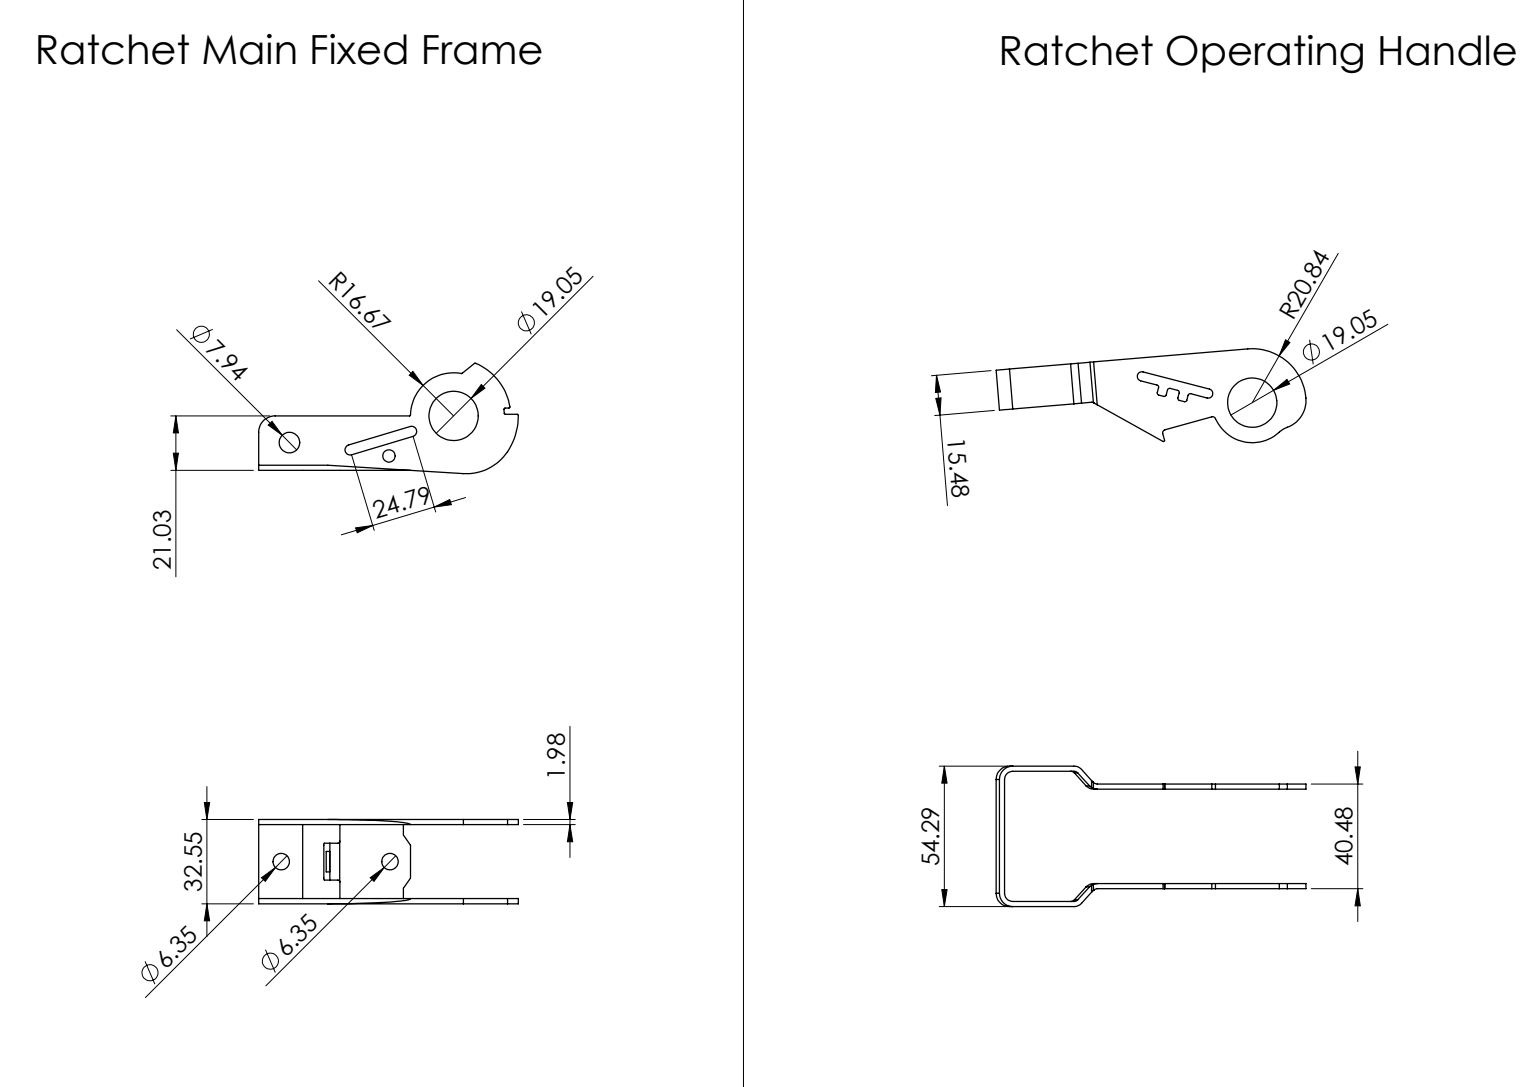
ISO-10303-21;
HEADER;
FILE_DESCRIPTION (('STEP AP214'),
    '1' );
FILE_NAME ('Ratchet Operating Handle.step',
    '2026-10-09T14:10:49',
    ( '' ),
    ( '' ),
    'SwSTEP 2.0',
    'SolidWorks 2026',
    '' );
FILE_SCHEMA (( 'AUTOMOTIVE_DESIGN' ));
ENDSEC;

DATA;
#1=VERTEX_POINT ( 'NONE', #18707 ) ;
#21=PLANE ( 'NONE',  #4977 ) ;
#37=EDGE_CURVE ( 'NONE', #10557, #1153, #11768, .T. ) ;
#54=VECTOR ( 'NONE', #11480, 1000.000000000000000 ) ;
#57=VECTOR ( 'NONE', #329, 1000.000000000000114 ) ;
#69=DIRECTION ( 'NONE',  ( -0.000000000000000000, -1.000000000000000000, 0.000000000000000000 ) ) ;
#81=LINE ( 'NONE', #19981, #4674 ) ;
#82=CARTESIAN_POINT ( 'NONE',  ( 29.01020070778135818, -3.968114999999999615, -13.85841188422236492 ) ) ;
#84=DIRECTION ( 'NONE',  ( 0.000000000000000000, 1.000000000000000000, 0.000000000000000000 ) ) ;
#85=CARTESIAN_POINT ( 'NONE',  ( -47.86112874365709047, 43.41875999999999891, -23.29368419115692035 ) ) ;
#88=ADVANCED_FACE ( 'NONE', ( #14317 ), #12096, .F. ) ;
#113=EDGE_LOOP ( 'NONE', ( #12441, #427, #14936, #388, #14608 ) ) ;
#128=VECTOR ( 'NONE', #842, 1000.000000000000000 ) ;
#135=VECTOR ( 'NONE', #21119, 1000.000000000000000 ) ;
#136=CARTESIAN_POINT ( 'NONE',  ( 20.56513292926062775, -14.84248999999999974, -10.49765270116350280 ) ) ;
#144=LINE ( 'NONE', #10317, #14114 ) ;
#149=EDGE_CURVE ( 'NONE', #1153, #19768, #10533, .T. ) ;
#153=VECTOR ( 'NONE', #12221, 1000.000000000000114 ) ;
#171=VERTEX_POINT ( 'NONE', #19036 ) ;
#172=DIRECTION ( 'NONE',  ( 0.000000000000000000, 1.000000000000000000, 0.000000000000000000 ) ) ;
#178=ORIENTED_EDGE ( 'NONE', *, *, #11385, .F. ) ;
#179=DIRECTION ( 'NONE',  ( -0.2490110332224836354, 0.000000000000000000, 0.9685006480810794960 ) ) ;
#193=( NAMED_UNIT ( * ) PLANE_ANGLE_UNIT ( ) SI_UNIT ( $, .RADIAN. ) );
#201=LINE ( 'NONE', #6943, #11370 ) ;
#211=ADVANCED_FACE ( 'NONE', ( #17509 ), #9084, .T. ) ;
#212=EDGE_CURVE ( 'NONE', #18633, #13378, #14563, .T. ) ;
#216=CARTESIAN_POINT ( 'NONE',  ( 19.79515554403045741, -1.983739999999999393, -10.69562145279641996 ) ) ;
#227=VERTEX_POINT ( 'NONE', #17942 ) ;
#236=CARTESIAN_POINT ( 'NONE',  ( -24.21104940531825633, 39.44874000000000080, -25.29232732678598339 ) ) ;
#246=CYLINDRICAL_SURFACE ( 'NONE', #5483, 3.970019999999997662 ) ;
#254=DIRECTION ( 'NONE',  ( -0.000000000000000000, -1.000000000000000000, 0.000000000000000000 ) ) ;
#255=PLANE ( 'NONE',  #7057 ) ;
#256=ORIENTED_EDGE ( 'NONE', *, *, #13831, .T. ) ;
#258=CARTESIAN_POINT ( 'NONE',  ( -13.87747867115857936, -3.968114999999999615, -9.458632424640695646 ) ) ;
#269=DIRECTION ( 'NONE',  ( -0.9685006480810792739, 0.000000000000000000, -0.2490110332224846346 ) ) ;
#276=EDGE_LOOP ( 'NONE', ( #21374, #11121, #4887, #17818 ) ) ;
#277=DIRECTION ( 'NONE',  ( 0.9964481331860212121, 0.000000000000000000, -0.08420877549337300871 ) ) ;
#283=DIRECTION ( 'NONE',  ( 0.7334850928793773539, -0.6768732144311023768, -0.06198604769976986950 ) ) ;
#287=CARTESIAN_POINT ( 'NONE',  ( 18.07371581377308800, 36.51313500000000545, -11.95909761906105473 ) ) ;
#296=CIRCLE ( 'NONE', #18309, 1.983739999999999393 ) ;
#298=DIRECTION ( 'NONE',  ( -0.4857267349359786768, 0.000000000000000000, 0.8741107132214052111 ) ) ;
#317=AXIS2_PLACEMENT_3D ( 'NONE', #448, #20660, #3437 ) ;
#329=DIRECTION ( 'NONE',  ( -0.9685006480810792739, 0.000000000000000000, -0.2490110332224846346 ) ) ;
#336=EDGE_CURVE ( 'NONE', #2732, #10479, #8823, .T. ) ;
#337=VERTEX_POINT ( 'NONE', #7187 ) ;
#338=CARTESIAN_POINT ( 'NONE',  ( -15.39353573898878658, -2.254660308866960339, -10.30107656633069979 ) ) ;
#339=EDGE_CURVE ( 'NONE', #11891, #20381, #4666, .T. ) ;
#345=DIRECTION ( 'NONE',  ( 0.000000000000000000, 1.000000000000000000, 0.000000000000000000 ) ) ;
#352=AXIS2_PLACEMENT_3D ( 'NONE', #14843, #6560, #1786 ) ;
#355=DIRECTION ( 'NONE',  ( 0.2490110332224846623, 0.000000000000000000, -0.9685006480810793850 ) ) ;
#358=CARTESIAN_POINT ( 'NONE',  ( 12.25799425556778388, 34.52875999999999834, 0.2069032437451798767 ) ) ;
#362=EDGE_CURVE ( 'NONE', #10171, #5161, #12705, .T. ) ;
#366=CARTESIAN_POINT ( 'NONE',  ( -53.00154558624916490, -5.714999999999999858, -22.85927301266823264 ) ) ;
#369=DIRECTION ( 'NONE',  ( -0.9964481331860212121, 0.000000000000000000, 0.08420877549337300871 ) ) ;
#374=VERTEX_POINT ( 'NONE', #3870 ) ;
#382=VECTOR ( 'NONE', #11141, 1000.000000000000000 ) ;
#383=CARTESIAN_POINT ( 'NONE',  ( 17.10576967688479399, -14.84248999999999974, -11.38708898545455561 ) ) ;
#385=ORIENTED_EDGE ( 'NONE', *, *, #5454, .T. ) ;
#388=ORIENTED_EDGE ( 'NONE', *, *, #17748, .F. ) ;
#397=AXIS2_PLACEMENT_3D ( 'NONE', #13888, #8758, #15657 ) ;
#398=DIRECTION ( 'NONE',  ( 0.4857267349359797870, 0.000000000000000000, -0.8741107132214044340 ) ) ;
#403=CARTESIAN_POINT ( 'NONE',  ( 29.45491884992628329, 34.52875999999999834, -15.58809351040512325 ) ) ;
#407=VECTOR ( 'NONE', #5440, 1000.000000000000000 ) ;
#414=CARTESIAN_POINT ( 'NONE',  ( 17.22522857595987844, 34.52875999999999834, -15.04442098945225403 ) ) ;
#422=AXIS2_PLACEMENT_3D ( 'NONE', #16207, #16521, #8217 ) ;
#427=ORIENTED_EDGE ( 'NONE', *, *, #17403, .F. ) ;
#428=ORIENTED_EDGE ( 'NONE', *, *, #17879, .F. ) ;
#437=EDGE_CURVE ( 'NONE', #16850, #6939, #17013, .T. ) ;
#438=CARTESIAN_POINT ( 'NONE',  ( 31.83819605565793509, 34.52875999999999834, -4.158220719828246814 ) ) ;
#443=ORIENTED_EDGE ( 'NONE', *, *, #13997, .T. ) ;
#445=CARTESIAN_POINT ( 'NONE',  ( 17.87574706213523612, -3.968114999999999615, -11.18912023382283571 ) ) ;
#446=DIRECTION ( 'NONE',  ( -0.2490110332224846346, 0.000000000000000000, 0.9685006480810792739 ) ) ;
#448=CARTESIAN_POINT ( 'NONE',  ( 55.81697695389291169, -14.84248999999999974, -11.14520323105768362 ) ) ;
#451=ADVANCED_FACE ( 'NONE', ( #15819 ), #9149, .F. ) ;
#458=ORIENTED_EDGE ( 'NONE', *, *, #17617, .T. ) ;
#460=CARTESIAN_POINT ( 'NONE',  ( -15.84035234298960049, -2.442431200715369677, -10.46642885967791692 ) ) ;
#464=CARTESIAN_POINT ( 'NONE',  ( 11.56192577415882816, -1.983739999999999393, 4.677561850332325299 ) ) ;
#466=DIRECTION ( 'NONE',  ( -0.4857267349359799535, 0.000000000000000000, 0.8741107132214044340 ) ) ;
#471=PRODUCT_DEFINITION ( 'UNKNOWN', '', #9128, #21835 ) ;
#487=DIRECTION ( 'NONE',  ( -0.2490110332224846346, 0.000000000000000000, 0.9685006480810792739 ) ) ;
#488=AXIS2_PLACEMENT_3D ( 'NONE', #287, #69, #10464 ) ;
#489=DIRECTION ( 'NONE',  ( -0.9685006480810794960, 0.000000000000000000, -0.2490110332224836354 ) ) ;
#496=EDGE_CURVE ( 'NONE', #17843, #3371, #1299, .T. ) ;
#519=ADVANCED_FACE ( 'NONE', ( #14481 ), #16142, .F. ) ;
#520=CARTESIAN_POINT ( 'NONE',  ( 46.03750000000000142, -14.84248999999999974, -10.31874999999999964 ) ) ;
#534=DIRECTION ( 'NONE',  ( 0.7334850928793772429, -0.6768732144311024879, -0.06198604769977036216 ) ) ;
#545=CARTESIAN_POINT ( 'NONE',  ( 46.03750000000000142, -3.968114999999999615, -10.31874999999999964 ) ) ;
#549=ORIENTED_EDGE ( 'NONE', *, *, #989, .F. ) ;
#552=LINE ( 'NONE', #7622, #13154 ) ;
#555=DIRECTION ( 'NONE',  ( 0.000000000000000000, 1.000000000000000000, 0.000000000000000000 ) ) ;
#556=ADVANCED_FACE ( 'NONE', ( #9374 ), #2746, .T. ) ;
#558=ORIENTED_EDGE ( 'NONE', *, *, #17949, .F. ) ;
#561=CARTESIAN_POINT ( 'NONE',  ( 22.02657784715807665, 128.5105379999999968, -12.98906981665815330 ) ) ;
#579=DIRECTION ( 'NONE',  ( -0.9964481331860213231, 0.000000000000000000, 0.08420877549337293932 ) ) ;
#586=ORIENTED_EDGE ( 'NONE', *, *, #10826, .T. ) ;
#590=ORIENTED_EDGE ( 'NONE', *, *, #21010, .F. ) ;
#595=ORIENTED_EDGE ( 'NONE', *, *, #11225, .F. ) ;
#601=FACE_OUTER_BOUND ( 'NONE', #956, .T. ) ;
#605=ORIENTED_EDGE ( 'NONE', *, *, #6499, .F. ) ;
#608=DIRECTION ( 'NONE',  ( 0.08420877549337300871, 0.000000000000000000, 0.9964481331860212121 ) ) ;
#612=CARTESIAN_POINT ( 'NONE',  ( 3.805353748838121053, -1.983739999999999393, -22.18284873352824960 ) ) ;
#615=ORIENTED_EDGE ( 'NONE', *, *, #14572, .T. ) ;
#618=ADVANCED_FACE ( 'NONE', ( #9701 ), #12829, .F. ) ;
#626=CARTESIAN_POINT ( 'NONE',  ( 17.99520596118501814, -14.84248999999999974, -14.84645223781840073 ) ) ;
#627=FACE_OUTER_BOUND ( 'NONE', #9472, .T. ) ;
#639=EDGE_CURVE ( 'NONE', #5833, #5959, #21527, .T. ) ;
#649=CARTESIAN_POINT ( 'NONE',  ( 11.42842559562532578, -3.968114999999999615, 1.673196738795719174 ) ) ;
#657=ORIENTED_EDGE ( 'NONE', *, *, #6799, .T. ) ;
#660=DIRECTION ( 'NONE',  ( 0.2490110332224846346, 0.000000000000000000, -0.9685006480810792739 ) ) ;
#666=LINE ( 'NONE', #20779, #7420 ) ;
#674=EDGE_CURVE ( 'NONE', #1, #6701, #6424, .T. ) ;
#680=AXIS2_PLACEMENT_3D ( 'NONE', #2628, #20743, #5925 ) ;
#686=FACE_OUTER_BOUND ( 'NONE', #17221, .T. ) ;
#694=CARTESIAN_POINT ( 'NONE',  ( -16.14706788831979978, 36.51313500000000545, -25.97380585690919830 ) ) ;
#698=CARTESIAN_POINT ( 'NONE',  ( 28.56548256563643662, -14.84248999999999974, -12.12873025803960658 ) ) ;
#701=AXIS2_PLACEMENT_3D ( 'NONE', #14633, #10960, #2564 ) ;
#714=ORIENTED_EDGE ( 'NONE', *, *, #19357, .F. ) ;
#722=LINE ( 'NONE', #20832, #16647 ) ;
#725=CYLINDRICAL_SURFACE ( 'NONE', #8862, 20.83593749999999289 ) ;
#728=DIRECTION ( 'NONE',  ( 0.000000000000000000, 1.000000000000000000, 0.000000000000000000 ) ) ;
#737=CARTESIAN_POINT ( 'NONE',  ( -46.55773479047372376, 43.41875999999999891, -7.870535429687039120 ) ) ;
#740=ORIENTED_EDGE ( 'NONE', *, *, #20509, .F. ) ;
#742=VECTOR ( 'NONE', #16555, 1000.000000000000114 ) ;
#755=AXIS2_PLACEMENT_3D ( 'NONE', #8975, #21028, #5874 ) ;
#759=CYLINDRICAL_SURFACE ( 'NONE', #18143, 3.970019999999997662 ) ;
#779=ORIENTED_EDGE ( 'NONE', *, *, #14955, .F. ) ;
#785=CARTESIAN_POINT ( 'NONE',  ( 12.13621795668766445, 36.51313500000000545, 4.225309685850866082 ) ) ;
#800=PLANE ( 'NONE',  #15930 ) ;
#801=FACE_OUTER_BOUND ( 'NONE', #18130, .T. ) ;
#823=ADVANCED_FACE ( 'NONE', ( #18322 ), #1521, .F. ) ;
#828=ORIENTED_EDGE ( 'NONE', *, *, #12493, .F. ) ;
#842=DIRECTION ( 'NONE',  ( 0.000000000000000000, 1.000000000000000000, 0.000000000000000000 ) ) ;
#846=ORIENTED_EDGE ( 'NONE', *, *, #8565, .F. ) ;
#848=CARTESIAN_POINT ( 'NONE',  ( -15.27935546639805331, -3.968114999999999615, -26.04713531390440906 ) ) ;
#853=CARTESIAN_POINT ( 'NONE',  ( 21.25660046192028929, -3.968114999999999615, -13.18703856829094079 ) ) ;
#870=ORIENTED_EDGE ( 'NONE', *, *, #639, .T. ) ;
#882=EDGE_CURVE ( 'NONE', #20855, #10784, #15692, .T. ) ;
#889=ORIENTED_EDGE ( 'NONE', *, *, #967, .T. ) ;
#898=ADVANCED_FACE ( 'NONE', ( #17208 ), #2170, .T. ) ;
#899=ADVANCED_FACE ( 'NONE', ( #19304 ), #7270, .T. ) ;
#902=CARTESIAN_POINT ( 'NONE',  ( 62.90077106633562209, -1.983739999999999393, 8.141649473166729933 ) ) ;
#919=ORIENTED_EDGE ( 'NONE', *, *, #7931, .T. ) ;
#920=CARTESIAN_POINT ( 'NONE',  ( 12.57635667311951622, -95.96551800000000298, 1.354834321244424267 ) ) ;
#932=DIRECTION ( 'NONE',  ( 0.9964481331860212121, 0.000000000000000000, -0.08420877549337300871 ) ) ;
#945=ORIENTED_EDGE ( 'NONE', *, *, #5714, .F. ) ;
#950=VECTOR ( 'NONE', #4203, 1000.000000000000000 ) ;
#951=DIRECTION ( 'NONE',  ( 0.08420877549337300871, 0.000000000000000000, 0.9964481331860212121 ) ) ;
#952=ORIENTED_EDGE ( 'NONE', *, *, #8551, .F. ) ;
#956=EDGE_LOOP ( 'NONE', ( #8354, #9146, #16354, #4398, #16333 ) ) ;
#957=ORIENTED_EDGE ( 'NONE', *, *, #13068, .F. ) ;
#967=EDGE_CURVE ( 'NONE', #10206, #3833, #5592, .T. ) ;
#969=DIRECTION ( 'NONE',  ( 0.2490110332224846623, 0.000000000000000000, -0.9685006480810793850 ) ) ;
#972=DIRECTION ( 'NONE',  ( 0.08420877549337300871, 0.000000000000000000, 0.9964481331860212121 ) ) ;
#987=ORIENTED_EDGE ( 'NONE', *, *, #21537, .F. ) ;
#988=CARTESIAN_POINT ( 'NONE',  ( 21.25660046192028929, 36.51313500000000545, -13.18703856829094079 ) ) ;
#989=EDGE_CURVE ( 'NONE', #17468, #15052, #4063, .T. ) ;
#997=LINE ( 'NONE', #1322, #15546 ) ;
#1029=AXIS2_PLACEMENT_3D ( 'NONE', #3066, #20273, #16870 ) ;
#1037=ORIENTED_EDGE ( 'NONE', *, *, #13043, .F. ) ;
#1054=VERTEX_POINT ( 'NONE', #6558 ) ;
#1064=CARTESIAN_POINT ( 'NONE',  ( 22.02657784715807665, 128.5105379999999968, -12.98906981665815330 ) ) ;
#1066=PLANE ( 'NONE',  #17926 ) ;
#1079=AXIS2_PLACEMENT_3D ( 'NONE', #9658, #1255, #20244 ) ;
#1080=DIRECTION ( 'NONE',  ( -0.7334850928793776870, -0.6768732144311018217, 0.06198604769977172219 ) ) ;
#1083=DIRECTION ( 'NONE',  ( 0.9964481331860213231, 0.000000000000000000, -0.08420877549337293932 ) ) ;
#1098=CARTESIAN_POINT ( 'NONE',  ( 13.28822531734660828, -3.968114999999999615, -15.23578611614444078 ) ) ;
#1102=CIRCLE ( 'NONE', #15593, 1.785937499999998179 ) ;
#1109=AXIS2_PLACEMENT_3D ( 'NONE', #9708, #17905, #16474 ) ;
#1122=ORIENTED_EDGE ( 'NONE', *, *, #16792, .F. ) ;
#1148=CARTESIAN_POINT ( 'NONE',  ( 56.47666780297049627, -3.968114999999999615, 1.109116340531466127 ) ) ;
#1153=VERTEX_POINT ( 'NONE', #3359 ) ;
#1155=DIRECTION ( 'NONE',  ( -0.9964481331860213231, 0.000000000000000000, 0.08420877549337311974 ) ) ;
#1178=VECTOR ( 'NONE', #4215, 1000.000000000000000 ) ;
#1189=CIRCLE ( 'NONE', #7538, 0.3962399999999998701 ) ;
#1203=DIRECTION ( 'NONE',  ( 0.2672484743474500268, 0.000000000000000000, 0.9636276526537417286 ) ) ;
#1205=CARTESIAN_POINT ( 'NONE',  ( 56.47666780297049627, -3.968114999999999615, 1.109116340531466127 ) ) ;
#1213=AXIS2_PLACEMENT_3D ( 'NONE', #19754, #4306, #16360 ) ;
#1230=LINE ( 'NONE', #7973, #13495 ) ;
#1238=VERTEX_POINT ( 'NONE', #1148 ) ;
#1246=CARTESIAN_POINT ( 'NONE',  ( 11.56192577415882816, 36.51313500000000545, 4.677561850332325299 ) ) ;
#1255=DIRECTION ( 'NONE',  ( 0.000000000000000000, -1.000000000000000000, 0.000000000000000000 ) ) ;
#1259=FACE_OUTER_BOUND ( 'NONE', #19368, .T. ) ;
#1270=ORIENTED_EDGE ( 'NONE', *, *, #10185, .T. ) ;
#1274=ORIENTED_EDGE ( 'NONE', *, *, #7778, .T. ) ;
#1297=CIRCLE ( 'NONE', #8709, 9.524999999999996803 ) ;
#1298=VERTEX_POINT ( 'NONE', #20448 ) ;
#1299=LINE ( 'NONE', #4515, #19490 ) ;
#1300=CARTESIAN_POINT ( 'NONE',  ( 3.360635606688116894, -14.84248999999999974, -20.45316710734507026 ) ) ;
#1309=CARTESIAN_POINT ( 'NONE',  ( 44.28293121686854761, -14.84248999999999974, -31.08068102505560759 ) ) ;
#1310=ORIENTED_EDGE ( 'NONE', *, *, #6278, .F. ) ;
#1314=VECTOR ( 'NONE', #9026, 1000.000000000000000 ) ;
#1318=EDGE_LOOP ( 'NONE', ( #8163, #16401, #5359, #8233 ) ) ;
#1322=CARTESIAN_POINT ( 'NONE',  ( 66.79943102505561114, 34.52875999999999834, -12.07331878313145168 ) ) ;
#1324=DIRECTION ( 'NONE',  ( -0.3447671952293630548, 0.000000000000000000, -0.9386882235831439658 ) ) ;
#1334=CARTESIAN_POINT ( 'NONE',  ( 11.82678039945931481, 34.52875999999999834, -12.74436900065013667 ) ) ;
#1339=ORIENTED_EDGE ( 'NONE', *, *, #14024, .F. ) ;
#1352=PLANE ( 'NONE',  #4444 ) ;
#1354=LINE ( 'NONE', #4474, #2136 ) ;
#1359=AXIS2_PLACEMENT_3D ( 'NONE', #18822, #254, #8753 ) ;
#1360=ORIENTED_EDGE ( 'NONE', *, *, #4217, .F. ) ;
#1367=ORIENTED_EDGE ( 'NONE', *, *, #16026, .F. ) ;
#1375=VERTEX_POINT ( 'NONE', #7425 ) ;
#1377=ADVANCED_FACE ( 'NONE', ( #19255 ), #5657, .F. ) ;
#1391=ORIENTED_EDGE ( 'NONE', *, *, #17921, .T. ) ;
#1392=CARTESIAN_POINT ( 'NONE',  ( 20.56513292926062775, -14.84248999999999974, -10.49765270116350280 ) ) ;
#1397=CIRCLE ( 'NONE', #21171, 0.7950200000000000600 ) ;
#1426=EDGE_LOOP ( 'NONE', ( #6037, #3965, #6020, #16638 ) ) ;
#1431=ADVANCED_FACE ( 'NONE', ( #7647 ), #14408, .T. ) ;
#1434=VECTOR ( 'NONE', #1830, 1000.000000000000114 ) ;
#1444=CARTESIAN_POINT ( 'NONE',  ( 12.13621795668766445, -3.968114999999999615, 4.225309685850866082 ) ) ;
#1447=CARTESIAN_POINT ( 'NONE',  ( -51.84716326864270286, -5.714364999999999029, -70.46824097531958842 ) ) ;
#1460=EDGE_CURVE ( 'NONE', #20489, #19935, #16020, .T. ) ;
#1468=DIRECTION ( 'NONE',  ( 0.2490110332224846623, 0.000000000000000000, -0.9685006480810793850 ) ) ;
#1478=DIRECTION ( 'NONE',  ( -0.9964481331860212121, 0.000000000000000000, 0.08420877549337300871 ) ) ;
#1490=ORIENTED_EDGE ( 'NONE', *, *, #10715, .F. ) ;
#1517=ADVANCED_FACE ( 'NONE', ( #19873 ), #19758, .T. ) ;
#1521=PLANE ( 'NONE',  #18095 ) ;
#1525=VERTEX_POINT ( 'NONE', #18125 ) ;
#1526=FACE_OUTER_BOUND ( 'NONE', #18731, .T. ) ;
#1530=VECTOR ( 'NONE', #12478, 1000.000000000000114 ) ;
#1532=ORIENTED_EDGE ( 'NONE', *, *, #17236, .T. ) ;
#1540=AXIS2_PLACEMENT_3D ( 'NONE', #3782, #466, #5769 ) ;
#1558=LINE ( 'NONE', #4877, #10288 ) ;
#1563=EDGE_CURVE ( 'NONE', #1054, #8841, #14380, .T. ) ;
#1564=EDGE_CURVE ( 'NONE', #21044, #4458, #13163, .T. ) ;
#1569=CARTESIAN_POINT ( 'NONE',  ( -15.39353573898878658, 34.79968030885680008, -10.30107656633069979 ) ) ;
#1570=AXIS2_PLACEMENT_3D ( 'NONE', #3806, #14001, #17411 ) ;
#1581=DIRECTION ( 'NONE',  ( -0.9685006480810793850, 0.000000000000000000, -0.2490110332224846623 ) ) ;
#1587=EDGE_CURVE ( 'NONE', #5833, #21613, #9486, .T. ) ;
#1622=VERTEX_POINT ( 'NONE', #21317 ) ;
#1624=DIRECTION ( 'NONE',  ( 0.000000000000000000, 1.000000000000000000, 0.000000000000000000 ) ) ;
#1630=LINE ( 'NONE', #8478, #12784 ) ;
#1631=PLANE ( 'NONE',  #5961 ) ;
#1633=ORIENTED_EDGE ( 'NONE', *, *, #15870, .F. ) ;
#1637=ORIENTED_EDGE ( 'NONE', *, *, #6499, .T. ) ;
#1638=ORIENTED_EDGE ( 'NONE', *, *, #8866, .F. ) ;
#1652=FACE_OUTER_BOUND ( 'NONE', #18846, .T. ) ;
#1657=EDGE_CURVE ( 'NONE', #8399, #20861, #20397, .T. ) ;
#1660=DIRECTION ( 'NONE',  ( 0.08420877549337300871, 0.000000000000000000, 0.9964481331860212121 ) ) ;
#1662=ORIENTED_EDGE ( 'NONE', *, *, #3097, .T. ) ;
#1667=AXIS2_PLACEMENT_3D ( 'NONE', #11026, #9465, #4401 ) ;
#1676=DIRECTION ( 'NONE',  ( 0.9685006480810793850, 0.000000000000000000, 0.2490110332224846623 ) ) ;
#1692=LINE ( 'NONE', #3473, #20854 ) ;
#1712=CARTESIAN_POINT ( 'NONE',  ( -15.41509608936259035, -4.609114529603660415, -10.31276839742836415 ) ) ;
#1715=VERTEX_POINT ( 'NONE', #6720 ) ;
#1730=CARTESIAN_POINT ( 'NONE',  ( -14.90829243662735060, -2.075094819660129986, -10.03143607188699526 ) ) ;
#1754=DIRECTION ( 'NONE',  ( 0.000000000000000000, 1.000000000000000000, 0.000000000000000000 ) ) ;
#1759=DIRECTION ( 'NONE',  ( -0.000000000000000000, -1.000000000000000000, 0.000000000000000000 ) ) ;
#1761=LINE ( 'NONE', #8507, #17257 ) ;
#1779=ADVANCED_FACE ( 'NONE', ( #1526 ), #8369, .F. ) ;
#1780=AXIS2_PLACEMENT_3D ( 'NONE', #17428, #17535, #277 ) ;
#1786=DIRECTION ( 'NONE',  ( 0.9685006480810794960, 0.000000000000000000, 0.2490110332224836354 ) ) ;
#1800=CARTESIAN_POINT ( 'NONE',  ( 3.805353748838121053, -14.84248999999999974, -22.18284873352824960 ) ) ;
#1815=VECTOR ( 'NONE', #20879, 1000.000000000000000 ) ;
#1824=EDGE_LOOP ( 'NONE', ( #17987, #8783, #945, #11646 ) ) ;
#1826=CIRCLE ( 'NONE', #21612, 9.524999999999996803 ) ;
#1830=DIRECTION ( 'NONE',  ( -0.9685006480810792739, 0.000000000000000000, -0.2490110332224846346 ) ) ;
#1835=VECTOR ( 'NONE', #1851, 1000.000000000000114 ) ;
#1836=CARTESIAN_POINT ( 'NONE',  ( 3.805353748838121053, 36.51313500000000545, -22.18284873352824960 ) ) ;
#1837=EDGE_CURVE ( 'NONE', #16799, #19840, #20975, .T. ) ;
#1846=CIRCLE ( 'NONE', #12107, 11.02160133116777985 ) ;
#1851=DIRECTION ( 'NONE',  ( -0.6744690509234934073, -0.7360996206939023345, 0.05699866455150641442 ) ) ;
#1852=SURFACE_STYLE_USAGE ( .BOTH. , #8477 ) ;
#1855=ORIENTED_EDGE ( 'NONE', *, *, #11172, .T. ) ;
#1860=ORIENTED_EDGE ( 'NONE', *, *, #496, .F. ) ;
#1861=AXIS2_PLACEMENT_3D ( 'NONE', #3512, #21650, #10140 ) ;
#1862=EDGE_LOOP ( 'NONE', ( #20036, #17938, #15260, #18256 ) ) ;
#1878=VECTOR ( 'NONE', #13860, 1000.000000000000000 ) ;
#1905=EDGE_CURVE ( 'NONE', #8949, #6182, #17556, .T. ) ;
#1911=CIRCLE ( 'NONE', #11461, 0.7950200000000003930 ) ;
#1924=EDGE_CURVE ( 'NONE', #19794, #14117, #13931, .T. ) ;
#1928=ORIENTED_EDGE ( 'NONE', *, *, #13864, .F. ) ;
#1932=EDGE_CURVE ( 'NONE', #19840, #9986, #12584, .T. ) ;
#1934=DIRECTION ( 'NONE',  ( -0.4857267349359786768, 0.000000000000000000, 0.8741107132214052111 ) ) ;
#1937=DIRECTION ( 'NONE',  ( -0.2490110332224836354, 0.000000000000000000, 0.9685006480810794960 ) ) ;
#1944=AXIS2_PLACEMENT_3D ( 'NONE', #14933, #11374, #7828 ) ;
#1953=EDGE_CURVE ( 'NONE', #7817, #3064, #9657, .T. ) ;
#1961=ORIENTED_EDGE ( 'NONE', *, *, #6404, .T. ) ;
#1979=EDGE_CURVE ( 'NONE', #12265, #10693, #1189, .T. ) ;
#1985=DIRECTION ( 'NONE',  ( 0.9636276526537417286, 0.000000000000000000, -0.2672484743474500268 ) ) ;
#1988=DIRECTION ( 'NONE',  ( -0.9964481331860212121, 0.000000000000000000, 0.08420877549337302259 ) ) ;
#1997=FACE_OUTER_BOUND ( 'NONE', #4358, .T. ) ;
#2002=EDGE_CURVE ( 'NONE', #16776, #7796, #14035, .T. ) ;
#2005=FACE_OUTER_BOUND ( 'NONE', #18425, .T. ) ;
#2007=DIRECTION ( 'NONE',  ( 0.2490110332224846623, 0.000000000000000000, -0.9685006480810793850 ) ) ;
#2040=DIRECTION ( 'NONE',  ( 0.6744690509234934073, 0.7360996206939024455, -0.05699866455150642136 ) ) ;
#2057=EDGE_LOOP ( 'NONE', ( #21720, #14710, #21033, #18291 ) ) ;
#2060=SURFACE_STYLE_FILL_AREA ( #18872 ) ;
#2064=ORIENTED_EDGE ( 'NONE', *, *, #15467, .F. ) ;
#2080=EDGE_CURVE ( 'NONE', #3371, #8815, #17439, .T. ) ;
#2088=ORIENTED_EDGE ( 'NONE', *, *, #17214, .T. ) ;
#2090=LINE ( 'NONE', #20320, #5341 ) ;
#2094=DIRECTION ( 'NONE',  ( 0.9685006480810792739, 0.000000000000000000, 0.2490110332224846346 ) ) ;
#2102=AXIS2_PLACEMENT_3D ( 'NONE', #9867, #14883, #3257 ) ;
#2103=ADVANCED_FACE ( 'NONE', ( #21401 ), #21508, .T. ) ;
#2107=EDGE_CURVE ( 'NONE', #3226, #2636, #18100, .T. ) ;
#2109=DIRECTION ( 'NONE',  ( 0.9964481331860213231, 0.000000000000000000, -0.08420877549337293932 ) ) ;
#2129=ORIENTED_EDGE ( 'NONE', *, *, #10973, .F. ) ;
#2136=VECTOR ( 'NONE', #16627, 1000.000000000000000 ) ;
#2139=STYLED_ITEM ( 'NONE', ( #10043 ), #5939 ) ;
#2147=ORIENTED_EDGE ( 'NONE', *, *, #3587, .F. ) ;
#2160=ADVANCED_FACE ( 'NONE', ( #14464 ), #19532, .T. ) ;
#2170=CYLINDRICAL_SURFACE ( 'NONE', #16338, 15.47812499999999680 ) ;
#2177=CARTESIAN_POINT ( 'NONE',  ( 11.75439013559175017, 36.51313500000000545, 4.331204221326972359 ) ) ;
#2183=ORIENTED_EDGE ( 'NONE', *, *, #12051, .F. ) ;
#2184=AXIS2_PLACEMENT_3D ( 'NONE', #5383, #7375, #5600 ) ;
#2188=LINE ( 'NONE', #17454, #18085 ) ;
#2194=ORIENTED_EDGE ( 'NONE', *, *, #20013, .F. ) ;
#2201=CARTESIAN_POINT ( 'NONE',  ( -17.16618386210371483, 39.44874000000000080, 58.07004290071009223 ) ) ;
#2204=VERTEX_POINT ( 'NONE', #21073 ) ;
#2214=DIRECTION ( 'NONE',  ( -0.000000000000000000, -1.000000000000000000, 0.000000000000000000 ) ) ;
#2216=VERTEX_POINT ( 'NONE', #2729 ) ;
#2218=CIRCLE ( 'NONE', #18453, 3.970019999999998550 ) ;
#2233=VECTOR ( 'NONE', #21115, 1000.000000000000000 ) ;
#2234=AXIS2_PLACEMENT_3D ( 'NONE', #14022, #2275, #17644 ) ;
#2252=CYLINDRICAL_SURFACE ( 'NONE', #1570, 1.785937500000001510 ) ;
#2271=DIRECTION ( 'NONE',  ( -0.9685006480810794960, 0.000000000000000000, -0.2490110332224836354 ) ) ;
#2275=DIRECTION ( 'NONE',  ( 0.000000000000000000, 0.000000000000000000, 1.000000000000000000 ) ) ;
#2277=FACE_OUTER_BOUND ( 'NONE', #16147, .T. ) ;
#2281=ORIENTED_EDGE ( 'NONE', *, *, #19742, .F. ) ;
#2287=AXIS2_PLACEMENT_3D ( 'NONE', #20417, #1754, #4969 ) ;
#2288=EDGE_CURVE ( 'NONE', #1054, #20069, #12884, .T. ) ;
#2301=ORIENTED_EDGE ( 'NONE', *, *, #9369, .F. ) ;
#2305=ORIENTED_EDGE ( 'NONE', *, *, #3869, .F. ) ;
#2306=CARTESIAN_POINT ( 'NONE',  ( 12.13621795668766445, 36.51313500000000545, 4.225309685850866082 ) ) ;
#2316=CARTESIAN_POINT ( 'NONE',  ( 17.22522857595987844, -1.983739999999999393, -15.04442098945225403 ) ) ;
#2345=EDGE_CURVE ( 'NONE', #13041, #20031, #19352, .T. ) ;
#2349=DIRECTION ( 'NONE',  ( -0.000000000000000000, -1.000000000000000000, 0.000000000000000000 ) ) ;
#2381=EDGE_LOOP ( 'NONE', ( #6945, #15252, #13580, #3398 ) ) ;
#2393=EDGE_CURVE ( 'NONE', #21254, #13041, #13982, .T. ) ;
#2407=DIRECTION ( 'NONE',  ( -0.9964481331860212121, 0.000000000000000000, 0.08420877549337300871 ) ) ;
#2409=VERTEX_POINT ( 'NONE', #19252 ) ;
#2410=VECTOR ( 'NONE', #7152, 1000.000000000000114 ) ;
#2413=ORIENTED_EDGE ( 'NONE', *, *, #12523, .F. ) ;
#2422=CARTESIAN_POINT ( 'NONE',  ( -47.86112874365709047, -10.87373999999999974, -23.29368419115692035 ) ) ;
#2428=DIRECTION ( 'NONE',  ( 0.8741107132214044340, 0.000000000000000000, 0.4857267349359799535 ) ) ;
#2451=VECTOR ( 'NONE', #11304, 1000.000000000000114 ) ;
#2459=DIRECTION ( 'NONE',  ( 0.2490110332224836354, 0.000000000000000000, -0.9685006480810794960 ) ) ;
#2463=AXIS2_PLACEMENT_3D ( 'NONE', #9443, #11327, #18078 ) ;
#2467=CARTESIAN_POINT ( 'NONE',  ( -15.97216256926745714, -95.96551800000000298, -9.259783438096400587 ) ) ;
#2472=EDGE_CURVE ( 'NONE', #9581, #2549, #6850, .T. ) ;
#2473=ADVANCED_FACE ( 'NONE', ( #7749, #3101, #8066 ), #14631, .F. ) ;
#2474=CARTESIAN_POINT ( 'NONE',  ( 20.76310168089343478, 34.52875999999999834, -11.26763008640078212 ) ) ;
#2489=ORIENTED_EDGE ( 'NONE', *, *, #16116, .F. ) ;
#2491=DIRECTION ( 'NONE',  ( 0.2490110332224846346, 0.000000000000000000, -0.9685006480810792739 ) ) ;
#2501=VECTOR ( 'NONE', #21012, 1000.000000000000000 ) ;
#2503=ORIENTED_EDGE ( 'NONE', *, *, #5945, .T. ) ;
#2507=DIRECTION ( 'NONE',  ( 0.000000000000000000, 1.000000000000000000, 0.000000000000000000 ) ) ;
#2508=DIRECTION ( 'NONE',  ( 0.000000000000000000, 1.000000000000000000, 0.000000000000000000 ) ) ;
#2513=CARTESIAN_POINT ( 'NONE',  ( 2.915917464538113180, 34.52875999999999834, -18.72348548116188027 ) ) ;
#2516=EDGE_CURVE ( 'NONE', #20607, #8815, #16278, .T. ) ;
#2518=EDGE_CURVE ( 'NONE', #2409, #12158, #4374, .T. ) ;
#2543=EDGE_CURVE ( 'NONE', #10465, #9581, #14404, .T. ) ;
#2549=VERTEX_POINT ( 'NONE', #11074 ) ;
#2563=DIRECTION ( 'NONE',  ( 0.08420877549337300871, 0.000000000000000000, 0.9964481331860212121 ) ) ;
#2564=DIRECTION ( 'NONE',  ( 0.000000000000000000, 1.000000000000000000, 0.000000000000000000 ) ) ;
#2574=EDGE_CURVE ( 'NONE', #6701, #19617, #20416, .T. ) ;
#2586=PLANE ( 'NONE',  #16764 ) ;
#2592=CARTESIAN_POINT ( 'NONE',  ( 31.83819605565793509, -1.983739999999999393, -4.158220719828246814 ) ) ;
#2596=AXIS2_PLACEMENT_3D ( 'NONE', #1064, #6365, #13028 ) ;
#2601=DIRECTION ( 'NONE',  ( -0.9685006480810794960, 0.000000000000000000, -0.2490110332224836354 ) ) ;
#2614=CARTESIAN_POINT ( 'NONE',  ( -22.90765545213488963, 43.41875999999999891, -9.869178565316103047 ) ) ;
#2615=VECTOR ( 'NONE', #17712, 1000.000000000000000 ) ;
#2622=VECTOR ( 'NONE', #2563, 1000.000000000000000 ) ;
#2624=EDGE_CURVE ( 'NONE', #20381, #15906, #3647, .T. ) ;
#2628=CARTESIAN_POINT ( 'NONE',  ( 9.058884679750676128, -3.968114999999999615, -16.32319115207028659 ) ) ;
#2629=CARTESIAN_POINT ( 'NONE',  ( 19.79515554403045741, -3.968114999999999615, -10.69562145279641996 ) ) ;
#2630=AXIS2_PLACEMENT_3D ( 'NONE', #1300, #13045, #14375 ) ;
#2632=ORIENTED_EDGE ( 'NONE', *, *, #4378, .T. ) ;
#2633=CARTESIAN_POINT ( 'NONE',  ( -14.45909654372175090, 36.51313499999967860, -9.781826438796489498 ) ) ;
#2635=DIRECTION ( 'NONE',  ( 0.000000000000000000, 1.000000000000000000, 0.000000000000000000 ) ) ;
#2636=VERTEX_POINT ( 'NONE', #8612 ) ;
#2647=CARTESIAN_POINT ( 'NONE',  ( -46.55710204590916135, 41.43438499999999891, -7.870588902259476605 ) ) ;
#2682=CARTESIAN_POINT ( 'NONE',  ( -47.86049599909252805, 41.43438499999999891, -23.29373766372935961 ) ) ;
#2686=DIRECTION ( 'NONE',  ( 0.3447671952293626108, 0.000000000000000000, 0.9386882235831439658 ) ) ;
#2700=DIRECTION ( 'NONE',  ( 0.000000000000000000, 1.000000000000000000, 0.000000000000000000 ) ) ;
#2703=FACE_BOUND ( 'NONE', #11148, .T. ) ;
#2706=CARTESIAN_POINT ( 'NONE',  ( 17.30373842852263877, 36.51313500000000545, -12.15706637069277107 ) ) ;
#2713=DIRECTION ( 'NONE',  ( 0.000000000000000000, 1.000000000000000000, 0.000000000000000000 ) ) ;
#2720=EDGE_CURVE ( 'NONE', #13936, #5560, #17797, .T. ) ;
#2729=CARTESIAN_POINT ( 'NONE',  ( 14.25617145423489696, -3.968114999999999615, -15.80779474975094168 ) ) ;
#2731=VERTEX_POINT ( 'NONE', #13614 ) ;
#2732=VERTEX_POINT ( 'NONE', #20098 ) ;
#2745=EDGE_CURVE ( 'NONE', #18449, #5398, #21668, .T. ) ;
#2746=PLANE ( 'NONE',  #10678 ) ;
#2748=DIRECTION ( 'NONE',  ( 0.08420877549337300871, 0.000000000000000000, 0.9964481331860212121 ) ) ;
#2760=DIRECTION ( 'NONE',  ( 0.9964481331860213231, 0.000000000000000000, -0.08420877549337293932 ) ) ;
#2763=ORIENTED_EDGE ( 'NONE', *, *, #9397, .T. ) ;
#2766=CARTESIAN_POINT ( 'NONE',  ( 11.42842559562532578, -1.983739999999999393, 1.673196738795719174 ) ) ;
#2775=DIRECTION ( 'NONE',  ( -0.000000000000000000, -1.000000000000000000, 0.000000000000000000 ) ) ;
#2781=FACE_OUTER_BOUND ( 'NONE', #14172, .T. ) ;
#2783=ORIENTED_EDGE ( 'NONE', *, *, #20016, .T. ) ;
#2787=ORIENTED_EDGE ( 'NONE', *, *, #15032, .F. ) ;
#2808=DIRECTION ( 'NONE',  ( -0.2490110332224857170, 0.000000000000000000, 0.9685006480810790519 ) ) ;
#2811=ORIENTED_EDGE ( 'NONE', *, *, #1979, .T. ) ;
#2814=CARTESIAN_POINT ( 'NONE',  ( 11.56192577415882816, 36.51313500000000545, 4.677561850332325299 ) ) ;
#2826=VECTOR ( 'NONE', #20288, 1000.000000000000000 ) ;
#2839=PLANE ( 'NONE',  #19092 ) ;
#2852=ORIENTED_EDGE ( 'NONE', *, *, #13364, .T. ) ;
#2853=VECTOR ( 'NONE', #17639, 1000.000000000000114 ) ;
#2858=LINE ( 'NONE', #19869, #10037 ) ;
#2859=AXIS2_PLACEMENT_3D ( 'NONE', #17284, #18934, #5675 ) ;
#2860=CARTESIAN_POINT ( 'NONE',  ( -16.07247711516169275, -5.309201820043501385, -10.44681224123558039 ) ) ;
#2865=DIRECTION ( 'NONE',  ( 0.9636276526537417286, 0.000000000000000000, -0.2672484743474500268 ) ) ;
#2868=DIRECTION ( 'NONE',  ( 0.2490110332224848289, 0.000000000000000000, -0.9685006480810792739 ) ) ;
#2886=ADVANCED_FACE ( 'NONE', ( #20650 ), #759, .T. ) ;
#2887=CARTESIAN_POINT ( 'NONE',  ( -15.39353573898878658, 37.13217763270220217, -10.30107656633069979 ) ) ;
#2912=EDGE_CURVE ( 'NONE', #8949, #12158, #4083, .T. ) ;
#2924=AXIS2_PLACEMENT_3D ( 'NONE', #5577, #18953, #1934 ) ;
#2950=EDGE_CURVE ( 'NONE', #10465, #1238, #16741, .T. ) ;
#2957=CIRCLE ( 'NONE', #4723, 1.191259999999999319 ) ;
#2959=CARTESIAN_POINT ( 'NONE',  ( 36.54633153140315471, -14.84248999999999974, -9.516661413425623550 ) ) ;
#2961=ORIENTED_EDGE ( 'NONE', *, *, #17403, .T. ) ;
#2971=ORIENTED_EDGE ( 'NONE', *, *, #17802, .T. ) ;
#2984=CARTESIAN_POINT ( 'NONE',  ( -16.07247711516169275, -5.309201820043501385, -10.44681224123558039 ) ) ;
#2991=DIRECTION ( 'NONE',  ( 0.000000000000000000, 1.000000000000000000, 0.000000000000000000 ) ) ;
#3001=CARTESIAN_POINT ( 'NONE',  ( 3.360635606688116894, -3.968114999999999615, -20.45316710734507026 ) ) ;
#3008=DIRECTION ( 'NONE',  ( -0.9685006480810794960, 0.000000000000000000, -0.2490110332224836354 ) ) ;
#3010=AXIS2_PLACEMENT_3D ( 'NONE', #11862, #6884, #17164 ) ;
#3011=FACE_OUTER_BOUND ( 'NONE', #16940, .T. ) ;
#3013=DIRECTION ( 'NONE',  ( 0.9964481331860212121, 0.000000000000000000, -0.08420877549337300871 ) ) ;
#3020=EDGE_CURVE ( 'NONE', #3845, #9830, #9375, .T. ) ;
#3023=DIRECTION ( 'NONE',  ( 0.9173788132826626862, 0.000000000000000000, -0.3980152169705242216 ) ) ;
#3025=ADVANCED_FACE ( 'NONE', ( #21418 ), #19430, .F. ) ;
#3030=DIRECTION ( 'NONE',  ( 0.08420877549337300871, 0.000000000000000000, 0.9964481331860212121 ) ) ;
#3037=DIRECTION ( 'NONE',  ( 0.3447671952293626108, 0.000000000000000000, 0.9386882235831439658 ) ) ;
#3038=FACE_OUTER_BOUND ( 'NONE', #10072, .T. ) ;
#3046=ORIENTED_EDGE ( 'NONE', *, *, #2107, .F. ) ;
#3064=VERTEX_POINT ( 'NONE', #7616 ) ;
#3066=CARTESIAN_POINT ( 'NONE',  ( -22.90765545213488963, 39.44874000000000080, -9.869178565316103047 ) ) ;
#3078=ORIENTED_EDGE ( 'NONE', *, *, #2543, .T. ) ;
#3096=ORIENTED_EDGE ( 'NONE', *, *, #21078, .F. ) ;
#3097=EDGE_CURVE ( 'NONE', #17763, #15906, #13157, .T. ) ;
#3101=FACE_BOUND ( 'NONE', #14158, .T. ) ;
#3104=CARTESIAN_POINT ( 'NONE',  ( -51.84779601320726528, -5.714999999999999858, -70.46818750274715626 ) ) ;
#3105=ORIENTED_EDGE ( 'NONE', *, *, #10351, .F. ) ;
#3107=LINE ( 'NONE', #16714, #19112 ) ;
#3110=DIRECTION ( 'NONE',  ( 0.000000000000000000, 1.000000000000000000, 0.000000000000000000 ) ) ;
#3116=EDGE_CURVE ( 'NONE', #7624, #6616, #2858, .T. ) ;
#3128=DIRECTION ( 'NONE',  ( 0.9964481331860213231, 0.000000000000000000, -0.08420877549337293932 ) ) ;
#3132=EDGE_CURVE ( 'NONE', #9903, #5598, #9324, .T. ) ;
#3138=VECTOR ( 'NONE', #10654, 1000.000000000000000 ) ;
#3146=CARTESIAN_POINT ( 'NONE',  ( 17.22522857595987844, -1.983739999999999393, -15.04442098945225403 ) ) ;
#3148=CARTESIAN_POINT ( 'NONE',  ( -14.99341658050624027, -4.186290746340128877, -10.07873794320046912 ) ) ;
#3159=ORIENTED_EDGE ( 'NONE', *, *, #14297, .F. ) ;
#3164=ORIENTED_EDGE ( 'NONE', *, *, #5578, .T. ) ;
#3176=CARTESIAN_POINT ( 'NONE',  ( -51.02421882195815783, -5.714364999999999029, -23.02637480153789795 ) ) ;
#3177=ORIENTED_EDGE ( 'NONE', *, *, #3301, .T. ) ;
#3194=ORIENTED_EDGE ( 'NONE', *, *, #19561, .F. ) ;
#3200=ORIENTED_EDGE ( 'NONE', *, *, #13479, .F. ) ;
#3218=LINE ( 'NONE', #6862, #12803 ) ;
#3223=CYLINDRICAL_SURFACE ( 'NONE', #11355, 3.174999999999999822 ) ;
#3226=VERTEX_POINT ( 'NONE', #6905 ) ;
#3257=DIRECTION ( 'NONE',  ( 0.000000000000000000, 1.000000000000000000, 0.000000000000000000 ) ) ;
#3261=DIRECTION ( 'NONE',  ( 0.08420877549337300871, 0.000000000000000000, 0.9964481331860212121 ) ) ;
#3277=ADVANCED_FACE ( 'NONE', ( #13777 ), #3596, .T. ) ;
#3278=AXIS2_PLACEMENT_3D ( 'NONE', #626, #19199, #17553 ) ;
#3281=EDGE_LOOP ( 'NONE', ( #15040, #14651, #4050, #19861 ) ) ;
#3299=ORIENTED_EDGE ( 'NONE', *, *, #989, .T. ) ;
#3301=EDGE_CURVE ( 'NONE', #5598, #1715, #13903, .T. ) ;
#3303=( GEOMETRIC_REPRESENTATION_CONTEXT ( 3 ) GLOBAL_UNCERTAINTY_ASSIGNED_CONTEXT ( ( #10781 ) ) GLOBAL_UNIT_ASSIGNED_CONTEXT ( ( #3721, #20834, #13917 ) ) REPRESENTATION_CONTEXT ( 'NONE', 'WORKASPACE' ) );
#3312=CARTESIAN_POINT ( 'NONE',  ( -15.39353573898878658, -4.587157632697119958, -10.30107656633069979 ) ) ;
#3317=CARTESIAN_POINT ( 'NONE',  ( 22.22454659879084460, 36.51313500000000545, -13.75904720189594244 ) ) ;
#3345=DIRECTION ( 'NONE',  ( 0.6744690509234934073, 0.7360996206939023345, -0.05699866455150641442 ) ) ;
#3352=CIRCLE ( 'NONE', #4412, 0.7950200000000000600 ) ;
#3355=AXIS2_PLACEMENT_3D ( 'NONE', #14168, #12500, #15603 ) ;
#3358=CARTESIAN_POINT ( 'NONE',  ( -53.00154558624916490, 38.26001999999999725, -22.85927301266823264 ) ) ;
#3359=CARTESIAN_POINT ( 'NONE',  ( 11.56192577415882816, -3.968114999999999615, 4.677561850332325299 ) ) ;
#3361=DIRECTION ( 'NONE',  ( 0.000000000000000000, 1.000000000000000000, 0.000000000000000000 ) ) ;
#3364=VERTEX_POINT ( 'NONE', #20817 ) ;
#3371=VERTEX_POINT ( 'NONE', #17855 ) ;
#3385=ORIENTED_EDGE ( 'NONE', *, *, #14955, .T. ) ;
#3389=ORIENTED_EDGE ( 'NONE', *, *, #16792, .T. ) ;
#3395=ORIENTED_EDGE ( 'NONE', *, *, #11430, .F. ) ;
#3398=ORIENTED_EDGE ( 'NONE', *, *, #16484, .F. ) ;
#3404=CARTESIAN_POINT ( 'NONE',  ( 22.22454659879084460, 36.51313500000000545, -13.75904720189594244 ) ) ;
#3422=EDGE_CURVE ( 'NONE', #14476, #21616, #11099, .T. ) ;
#3429=CYLINDRICAL_SURFACE ( 'NONE', #20028, 0.7950200000000003930 ) ;
#3433=CARTESIAN_POINT ( 'NONE',  ( 13.48619406898445661, -14.84248999999999974, -16.00576350138265624 ) ) ;
#3437=DIRECTION ( 'NONE',  ( -0.9964481331860213231, 0.000000000000000000, 0.08420877549337306422 ) ) ;
#3440=CARTESIAN_POINT ( 'NONE',  ( -49.72082486877479113, -5.714364999999999029, -7.603226040068017610 ) ) ;
#3442=ORIENTED_EDGE ( 'NONE', *, *, #16622, .F. ) ;
#3472=ORIENTED_EDGE ( 'NONE', *, *, #8565, .T. ) ;
#3473=CARTESIAN_POINT ( 'NONE',  ( -22.90765545213488963, -10.87373999999999974, -9.869178565316103047 ) ) ;
#3476=AXIS2_PLACEMENT_3D ( 'NONE', #14244, #16222, #14564 ) ;
#3498=FACE_OUTER_BOUND ( 'NONE', #3983, .T. ) ;
#3500=AXIS2_PLACEMENT_3D ( 'NONE', #7043, #8921, #15699 ) ;
#3503=AXIS2_PLACEMENT_3D ( 'NONE', #8893, #608, #21052 ) ;
#3506=CARTESIAN_POINT ( 'NONE',  ( -15.84345693979480352, 37.60427460010093625, -10.46616649349356365 ) ) ;
#3508=EDGE_CURVE ( 'NONE', #15795, #20381, #21264, .T. ) ;
#3512=CARTESIAN_POINT ( 'NONE',  ( 19.99312429566830218, -95.96551800000000298, -11.46559883803463720 ) ) ;
#3530=FACE_OUTER_BOUND ( 'NONE', #12817, .T. ) ;
#3542=ORIENTED_EDGE ( 'NONE', *, *, #14324, .F. ) ;
#3558=CARTESIAN_POINT ( 'NONE',  ( -15.60052840353448644, 34.87627845846405705, -10.41609846181108345 ) ) ;
#3568=DIRECTION ( 'NONE',  ( 0.08420877549337300871, 0.000000000000000000, 0.9964481331860212121 ) ) ;
#3570=AXIS2_PLACEMENT_3D ( 'NONE', #13020, #19952, #4600 ) ;
#3573=VECTOR ( 'NONE', #19065, 1000.000000000000000 ) ;
#3587=EDGE_CURVE ( 'NONE', #15164, #1238, #6869, .T. ) ;
#3596=PLANE ( 'NONE',  #16758 ) ;
#3602=ORIENTED_EDGE ( 'NONE', *, *, #7776, .T. ) ;
#3617=CARTESIAN_POINT ( 'NONE',  ( -47.86112874365709047, 38.26001999999999725, -23.29368419115692035 ) ) ;
#3622=DIRECTION ( 'NONE',  ( 0.8741107132214044340, 0.000000000000000000, 0.4857267349359799535 ) ) ;
#3632=ORIENTED_EDGE ( 'NONE', *, *, #15903, .T. ) ;
#3639=LINE ( 'NONE', #6946, #13108 ) ;
#3640=ORIENTED_EDGE ( 'NONE', *, *, #14297, .T. ) ;
#3643=AXIS2_PLACEMENT_3D ( 'NONE', #12774, #18270, #3128 ) ;
#3647=LINE ( 'NONE', #16707, #5422 ) ;
#3654=DIRECTION ( 'NONE',  ( 0.000000000000000000, 1.000000000000000000, 0.000000000000000000 ) ) ;
#3664=CARTESIAN_POINT ( 'NONE',  ( 14.25617145423489696, 36.51313500000000545, -15.80779474975094168 ) ) ;
#3673=CARTESIAN_POINT ( 'NONE',  ( 9.335363283976800375, -3.968114999999999615, -14.20581391854862474 ) ) ;
#3675=VECTOR ( 'NONE', #3945, 1000.000000000000000 ) ;
#3683=CARTESIAN_POINT ( 'NONE',  ( 28.56548256563643662, 36.51313500000000545, -12.12873025803960658 ) ) ;
#3686=CARTESIAN_POINT ( 'NONE',  ( 9.335363283976800375, -1.983739999999999393, -14.20581391854862474 ) ) ;
#3698=ADVANCED_FACE ( 'NONE', ( #5087 ), #18779, .F. ) ;
#3708=LINE ( 'NONE', #6802, #5999 ) ;
#3712=CIRCLE ( 'NONE', #17850, 0.7950200000000000600 ) ;
#3721=( LENGTH_UNIT ( ) NAMED_UNIT ( * ) SI_UNIT ( .MILLI., .METRE. ) );
#3722=EDGE_CURVE ( 'NONE', #8462, #9830, #12907, .T. ) ;
#3728=DIRECTION ( 'NONE',  ( 0.000000000000000000, 1.000000000000000000, 0.000000000000000000 ) ) ;
#3729=ORIENTED_EDGE ( 'NONE', *, *, #16884, .T. ) ;
#3739=DIRECTION ( 'NONE',  ( -0.9685006480810792739, 0.000000000000000000, -0.2490110332224846346 ) ) ;
#3745=ADVANCED_FACE ( 'NONE', ( #6955 ), #11934, .T. ) ;
#3746=ORIENTED_EDGE ( 'NONE', *, *, #18516, .F. ) ;
#3754=ORIENTED_EDGE ( 'NONE', *, *, #18480, .T. ) ;
#3768=DIRECTION ( 'NONE',  ( 0.000000000000000000, 1.000000000000000000, 0.000000000000000000 ) ) ;
#3769=FACE_OUTER_BOUND ( 'NONE', #14793, .T. ) ;
#3782=CARTESIAN_POINT ( 'NONE',  ( -15.71080452296940599, -14.84248999999999974, -10.47737680862620380 ) ) ;
#3783=FACE_OUTER_BOUND ( 'NONE', #21030, .T. ) ;
#3800=DIRECTION ( 'NONE',  ( 0.000000000000000000, 1.000000000000000000, 0.000000000000000000 ) ) ;
#3803=SHAPE_DEFINITION_REPRESENTATION ( #19043, #17083 ) ;
#3806=CARTESIAN_POINT ( 'NONE',  ( 29.01020070778135818, -14.84248999999999974, -13.85841188422236492 ) ) ;
#3807=ORIENTED_EDGE ( 'NONE', *, *, #2624, .T. ) ;
#3832=CIRCLE ( 'NONE', #14786, 0.7950200000000003930 ) ;
#3833=VERTEX_POINT ( 'NONE', #216 ) ;
#3841=CARTESIAN_POINT ( 'NONE',  ( 12.13621795668766445, 34.52875999999999834, 4.225309685850866082 ) ) ;
#3845=VERTEX_POINT ( 'NONE', #10392 ) ;
#3847=CARTESIAN_POINT ( 'NONE',  ( -21.45091887247874851, 40.79338547039380103, -9.992285829511605044 ) ) ;
#3852=ORIENTED_EDGE ( 'NONE', *, *, #18929, .F. ) ;
#3864=ORIENTED_EDGE ( 'NONE', *, *, #10321, .T. ) ;
#3867=EDGE_CURVE ( 'NONE', #8700, #18216, #8288, .T. ) ;
#3869=EDGE_CURVE ( 'NONE', #18216, #6968, #7191, .T. ) ;
#3870=CARTESIAN_POINT ( 'NONE',  ( -51.02421882195815783, -5.714364999999999029, -23.02637480153789795 ) ) ;
#3874=DIRECTION ( 'NONE',  ( -0.000000000000000000, -1.000000000000000000, 0.000000000000000000 ) ) ;
#3886=ORIENTED_EDGE ( 'NONE', *, *, #15205, .F. ) ;
#3893=LINE ( 'NONE', #15517, #1878 ) ;
#3906=CARTESIAN_POINT ( 'NONE',  ( 9.058884679750676128, 128.5105379999999968, -16.32319115207028659 ) ) ;
#3916=AXIS2_PLACEMENT_3D ( 'NONE', #4930, #11677, #8355 ) ;
#3929=UNCERTAINTY_MEASURE_WITH_UNIT (LENGTH_MEASURE( 1.000000000000000082E-05 ), #5164, 'distance_accuracy_value', 'NONE');
#3933=LINE ( 'NONE', #19058, #6323 ) ;
#3942=DIRECTION ( 'NONE',  ( -0.000000000000000000, -1.000000000000000000, 0.000000000000000000 ) ) ;
#3945=DIRECTION ( 'NONE',  ( -0.08420877549337300871, 0.000000000000000000, -0.9964481331860212121 ) ) ;
#3954=VECTOR ( 'NONE', #15173, 1000.000000000000114 ) ;
#3958=DIRECTION ( 'NONE',  ( -0.000000000000000000, -1.000000000000000000, 0.000000000000000000 ) ) ;
#3965=ORIENTED_EDGE ( 'NONE', *, *, #14127, .F. ) ;
#3968=ADVANCED_FACE ( 'NONE', ( #12386 ), #12270, .T. ) ;
#3972=AXIS2_PLACEMENT_3D ( 'NONE', #82, #12026, #20516 ) ;
#3976=VECTOR ( 'NONE', #15344, 1000.000000000000000 ) ;
#3979=CARTESIAN_POINT ( 'NONE',  ( -16.73439918454169018, 37.15413452960619622, -25.92417111164088084 ) ) ;
#3981=DIRECTION ( 'NONE',  ( 0.2490110332224846623, 0.000000000000000000, -0.9685006480810793850 ) ) ;
#3983=EDGE_LOOP ( 'NONE', ( #8656, #3299, #10213, #20181 ) ) ;
#3985=CARTESIAN_POINT ( 'NONE',  ( 9.335363283976800375, 34.52875999999999834, -14.20581391854862474 ) ) ;
#3986=LINE ( 'NONE', #5518, #8848 ) ;
#3987=FACE_OUTER_BOUND ( 'NONE', #5274, .T. ) ;
#3990=ORIENTED_EDGE ( 'NONE', *, *, #12213, .F. ) ;
#4005=AXIS2_PLACEMENT_3D ( 'NONE', #4522, #11259, #7725 ) ;
#4013=PLANE ( 'NONE',  #20830 ) ;
#4019=ADVANCED_FACE ( 'NONE', ( #15719 ), #19433, .F. ) ;
#4025=DIRECTION ( 'NONE',  ( 0.000000000000000000, 1.000000000000000000, 0.000000000000000000 ) ) ;
#4031=VERTEX_POINT ( 'NONE', #16044 ) ;
#4037=CYLINDRICAL_SURFACE ( 'NONE', #17325, 1.983739999999999393 ) ;
#4038=VERTEX_POINT ( 'NONE', #7618 ) ;
#4041=VECTOR ( 'NONE', #21286, 1000.000000000000000 ) ;
#4042=FACE_OUTER_BOUND ( 'NONE', #1426, .T. ) ;
#4044=EDGE_CURVE ( 'NONE', #20031, #14428, #17466, .T. ) ;
#4047=CARTESIAN_POINT ( 'NONE',  ( 66.79943102505561114, 36.51313500000000545, -12.07331878313145168 ) ) ;
#4050=ORIENTED_EDGE ( 'NONE', *, *, #14324, .T. ) ;
#4063=LINE ( 'NONE', #10805, #6788 ) ;
#4075=ORIENTED_EDGE ( 'NONE', *, *, #14515, .F. ) ;
#4079=CIRCLE ( 'NONE', #4436, 5.158740000000001658 ) ;
#4083=LINE ( 'NONE', #3979, #8596 ) ;
#4086=ORIENTED_EDGE ( 'NONE', *, *, #13438, .T. ) ;
#4088=LINE ( 'NONE', #2316, #16669 ) ;
#4109=DIRECTION ( 'NONE',  ( -0.9685006480810794960, 0.000000000000000000, -0.2490110332224836354 ) ) ;
#4121=EDGE_CURVE ( 'NONE', #8727, #20861, #19600, .T. ) ;
#4127=ORIENTED_EDGE ( 'NONE', *, *, #21754, .T. ) ;
#4141=EDGE_CURVE ( 'NONE', #16776, #1622, #4079, .T. ) ;
#4152=CARTESIAN_POINT ( 'NONE',  ( 22.02657784715807665, -1.983739999999999393, -12.98906981665815330 ) ) ;
#4161=VECTOR ( 'NONE', #7493, 1000.000000000000000 ) ;
#4167=DIRECTION ( 'NONE',  ( -0.9964481331860212121, 0.000000000000000000, 0.08420877549337300871 ) ) ;
#4174=ORIENTED_EDGE ( 'NONE', *, *, #19187, .F. ) ;
#4177=LINE ( 'NONE', #15923, #16631 ) ;
#4197=CARTESIAN_POINT ( 'NONE',  ( 3.805353748838121053, 34.52875999999999834, -22.18284873352824960 ) ) ;
#4199=ORIENTED_EDGE ( 'NONE', *, *, #3301, .F. ) ;
#4203=DIRECTION ( 'NONE',  ( -0.000000000000000000, -1.000000000000000000, 0.000000000000000000 ) ) ;
#4208=CARTESIAN_POINT ( 'NONE',  ( 29.45491884992628329, 36.51313500000000545, -15.58809351040512325 ) ) ;
#4215=DIRECTION ( 'NONE',  ( 0.08420877549337300871, 0.000000000000000000, 0.9964481331860212121 ) ) ;
#4217=EDGE_CURVE ( 'NONE', #14117, #20833, #5464, .T. ) ;
#4219=EDGE_CURVE ( 'NONE', #14428, #3833, #3712, .T. ) ;
#4220=PLANE ( 'NONE',  #701 ) ;
#4234=VECTOR ( 'NONE', #12383, 1000.000000000000000 ) ;
#4252=DIRECTION ( 'NONE',  ( 0.000000000000000000, 1.000000000000000000, 0.000000000000000000 ) ) ;
#4259=VERTEX_POINT ( 'NONE', #8689 ) ;
#4261=DIRECTION ( 'NONE',  ( -0.9964481331860211011, 0.000000000000000000, 0.08420877549337349444 ) ) ;
#4266=VERTEX_POINT ( 'NONE', #13587 ) ;
#4271=DIRECTION ( 'NONE',  ( 0.000000000000000000, 1.000000000000000000, 0.000000000000000000 ) ) ;
#4279=CARTESIAN_POINT ( 'NONE',  ( -22.90765545213488963, -10.87373999999999974, -9.869178565316103047 ) ) ;
#4284=DIRECTION ( 'NONE',  ( 0.000000000000000000, 1.000000000000000000, 0.000000000000000000 ) ) ;
#4288=ORIENTED_EDGE ( 'NONE', *, *, #12523, .T. ) ;
#4297=ORIENTED_EDGE ( 'NONE', *, *, #19624, .T. ) ;
#4298=EDGE_CURVE ( 'NONE', #21044, #12158, #13171, .T. ) ;
#4306=DIRECTION ( 'NONE',  ( 0.000000000000000000, 1.000000000000000000, 0.000000000000000000 ) ) ;
#4335=CARTESIAN_POINT ( 'NONE',  ( -16.73439918454169018, -4.609114529603660415, -25.92417111164088084 ) ) ;
#4338=DIRECTION ( 'NONE',  ( -0.000000000000000000, -1.000000000000000000, 0.000000000000000000 ) ) ;
#4354=FACE_OUTER_BOUND ( 'NONE', #12868, .T. ) ;
#4358=EDGE_LOOP ( 'NONE', ( #16778, #1037, #12724, #5122, #12340, #21411 ) ) ;
#4366=VECTOR ( 'NONE', #13807, 1000.000000000000000 ) ;
#4367=CARTESIAN_POINT ( 'NONE',  ( 17.22522857595987844, 36.51313500000000545, -15.04442098945225403 ) ) ;
#4372=EDGE_CURVE ( 'NONE', #16351, #21627, #12019, .T. ) ;
#4374=( BOUNDED_CURVE ( )  B_SPLINE_CURVE ( 3, ( #2887, #14734, #6414, #21440 ),
 .UNSPECIFIED., .F., .F. ) 
 B_SPLINE_CURVE_WITH_KNOTS ( ( 4, 4 ),
 ( 0.1347261119420776476, 0.1486429212228488894 ),
 .UNSPECIFIED. ) 
 CURVE ( )  GEOMETRIC_REPRESENTATION_ITEM ( )  RATIONAL_B_SPLINE_CURVE ( ( 1.000000000000000000, 0.9999838602667434628, 0.9999838602667434628, 1.000000000000000000 ) ) 
 REPRESENTATION_ITEM ( '' )  );
#4376=AXIS2_PLACEMENT_3D ( 'NONE', #5533, #17263, #2109 ) ;
#4378=EDGE_CURVE ( 'NONE', #20691, #5398, #18752, .T. ) ;
#4398=ORIENTED_EDGE ( 'NONE', *, *, #12330, .T. ) ;
#4401=DIRECTION ( 'NONE',  ( -0.9685006480810794960, 0.000000000000000000, -0.2490110332224836354 ) ) ;
#4412=AXIS2_PLACEMENT_3D ( 'NONE', #19274, #17516, #489 ) ;
#4417=EDGE_CURVE ( 'NONE', #19312, #21087, #5060, .T. ) ;
#4422=EDGE_CURVE ( 'NONE', #12648, #8841, #11812, .T. ) ;
#4425=DIRECTION ( 'NONE',  ( -0.6744690509234938514, 0.7360996206939018904, 0.05699866455150646993 ) ) ;
#4436=AXIS2_PLACEMENT_3D ( 'NONE', #9704, #13158, #7722 ) ;
#4437=ORIENTED_EDGE ( 'NONE', *, *, #1563, .T. ) ;
#4442=DIRECTION ( 'NONE',  ( 0.000000000000000000, 1.000000000000000000, 0.000000000000000000 ) ) ;
#4444=AXIS2_PLACEMENT_3D ( 'NONE', #8216, #1676, #1468 ) ;
#4445=CARTESIAN_POINT ( 'NONE',  ( 65.04486224192415023, 36.51313500000000545, -32.83524980818705785 ) ) ;
#4450=ORIENTED_EDGE ( 'NONE', *, *, #14838, .F. ) ;
#4453=DIRECTION ( 'NONE',  ( -0.9964481331860212121, 0.000000000000000000, 0.08420877549337300871 ) ) ;
#4458=VERTEX_POINT ( 'NONE', #16313 ) ;
#4474=CARTESIAN_POINT ( 'NONE',  ( 12.25799425556778388, 34.52875999999999834, 0.2069032437451798767 ) ) ;
#4494=EDGE_CURVE ( 'NONE', #6613, #13482, #9434, .T. ) ;
#4500=FACE_OUTER_BOUND ( 'NONE', #19320, .T. ) ;
#4505=DIRECTION ( 'NONE',  ( 0.000000000000000000, 1.000000000000000000, 0.000000000000000000 ) ) ;
#4515=CARTESIAN_POINT ( 'NONE',  ( 1.581041518826207692, -14.84248999999999974, -20.30277549736237575 ) ) ;
#4517=DIRECTION ( 'NONE',  ( 0.9964481331860212121, 0.000000000000000000, -0.08420877549337300871 ) ) ;
#4520=AXIS2_PLACEMENT_3D ( 'NONE', #20614, #5583, #398 ) ;
#4522=CARTESIAN_POINT ( 'NONE',  ( 46.03750000000000142, -1.983739999999999393, -10.31874999999999964 ) ) ;
#4525=DIRECTION ( 'NONE',  ( -0.000000000000000000, -1.000000000000000000, 0.000000000000000000 ) ) ;
#4542=DIRECTION ( 'NONE',  ( 0.000000000000000000, 1.000000000000000000, 0.000000000000000000 ) ) ;
#4550=CARTESIAN_POINT ( 'NONE',  ( 18.07371581377308800, -95.96551800000000298, -11.95909761906105473 ) ) ;
#4555=AXIS2_PLACEMENT_3D ( 'NONE', #12715, #16261, #11159 ) ;
#4561=CARTESIAN_POINT ( 'NONE',  ( 19.79515554403045741, -3.968114999999999615, -10.69562145279641996 ) ) ;
#4564=CARTESIAN_POINT ( 'NONE',  ( 22.22454659879084460, -3.968114999999999615, -13.75904720189594244 ) ) ;
#4567=DIRECTION ( 'NONE',  ( -0.8741107132214044340, 0.000000000000000000, -0.4857267349359799535 ) ) ;
#4577=FACE_OUTER_BOUND ( 'NONE', #13450, .T. ) ;
#4580=FACE_BOUND ( 'NONE', #15338, .T. ) ;
#4583=CARTESIAN_POINT ( 'NONE',  ( 9.058884679750676128, 36.51313500000000545, -16.32319115207028659 ) ) ;
#4586=LINE ( 'NONE', #7467, #6679 ) ;
#4600=DIRECTION ( 'NONE',  ( -0.2490110332224857170, 0.000000000000000000, 0.9685006480810790519 ) ) ;
#4610=ORIENTED_EDGE ( 'NONE', *, *, #3116, .T. ) ;
#4617=EDGE_CURVE ( 'NONE', #13996, #12465, #8794, .T. ) ;
#4639=EDGE_LOOP ( 'NONE', ( #9019, #17513, #15800, #10408 ) ) ;
#4653=FACE_BOUND ( 'NONE', #5476, .T. ) ;
#4664=ADVANCED_FACE ( 'NONE', ( #4577 ), #1352, .T. ) ;
#4666=CIRCLE ( 'NONE', #11019, 1.983739999999997838 ) ;
#4670=AXIS2_PLACEMENT_3D ( 'NONE', #10593, #7051, #534 ) ;
#4674=VECTOR ( 'NONE', #16688, 1000.000000000000114 ) ;
#4687=VECTOR ( 'NONE', #15000, 1000.000000000000114 ) ;
#4688=CIRCLE ( 'NONE', #17414, 1.983739999999999393 ) ;
#4695=CARTESIAN_POINT ( 'NONE',  ( 13.48619406898445661, -14.84248999999999974, -16.00576350138265624 ) ) ;
#4713=LINE ( 'NONE', #21170, #4041 ) ;
#4723=AXIS2_PLACEMENT_3D ( 'NONE', #8206, #14979, #6551 ) ;
#4727=ORIENTED_EDGE ( 'NONE', *, *, #5714, .T. ) ;
#4729=FACE_OUTER_BOUND ( 'NONE', #15220, .T. ) ;
#4734=AXIS2_PLACEMENT_3D ( 'NONE', #10494, #20536, #17240 ) ;
#4743=DIRECTION ( 'NONE',  ( -0.000000000000000000, -1.000000000000000000, 0.000000000000000000 ) ) ;
#4745=DIRECTION ( 'NONE',  ( -0.7334850928793775759, -0.6768732144311021548, 0.06198604769976992501 ) ) ;
#4749=CARTESIAN_POINT ( 'NONE',  ( -16.07247711516169275, 37.85422182005619618, -10.44681224123558039 ) ) ;
#4758=ORIENTED_EDGE ( 'NONE', *, *, #11943, .T. ) ;
#4778=PLANE ( 'NONE',  #10177 ) ;
#4779=ORIENTED_EDGE ( 'NONE', *, *, #11272, .F. ) ;
#4783=ORIENTED_EDGE ( 'NONE', *, *, #17214, .F. ) ;
#4788=DIRECTION ( 'NONE',  ( -0.2490110332224857170, 0.000000000000000000, 0.9685006480810790519 ) ) ;
#4794=B_SPLINE_CURVE_WITH_KNOTS ( 'NONE', 3,
 ( #20118, #5206, #3558, #1569 ),
 .UNSPECIFIED., .F., .F.,
 ( 4, 4 ),
 ( 0.000000000000000000, 1.000000000000000000 ),
 .UNSPECIFIED. ) ;
#4797=CARTESIAN_POINT ( 'NONE',  ( 17.30373842852263877, -3.968114999999999615, -12.15706637069277107 ) ) ;
#4803=CARTESIAN_POINT ( 'NONE',  ( -19.26602273594821924, -5.951855000000001006, -73.22163862549463431 ) ) ;
#4804=ORIENTED_EDGE ( 'NONE', *, *, #18929, .T. ) ;
#4805=DIRECTION ( 'NONE',  ( -0.000000000000000000, -1.000000000000000000, 0.000000000000000000 ) ) ;
#4808=ORIENTED_EDGE ( 'NONE', *, *, #19973, .F. ) ;
#4815=EDGE_LOOP ( 'NONE', ( #20974, #6268, #21494, #3864 ) ) ;
#4821=ADVANCED_FACE ( 'NONE', ( #8530 ), #20575, .T. ) ;
#4838=ORIENTED_EDGE ( 'NONE', *, *, #16622, .T. ) ;
#4841=EDGE_LOOP ( 'NONE', ( #17483, #13258, #15873, #9423 ) ) ;
#4847=CARTESIAN_POINT ( 'NONE',  ( 10.10534066920194185, 36.51313500000000545, -14.00784516691476966 ) ) ;
#4852=LINE ( 'NONE', #5163, #1835 ) ;
#4865=ADVANCED_FACE ( 'NONE', ( #10644 ), #18921, .T. ) ;
#4869=CARTESIAN_POINT ( 'NONE',  ( 30.42699695299585017, -1.983739999999999393, -4.832012189960551041 ) ) ;
#4875=EDGE_LOOP ( 'NONE', ( #20200, #15586, #17023, #4437 ) ) ;
#4877=CARTESIAN_POINT ( 'NONE',  ( 17.30373842852263877, -1.983739999999999393, -12.15706637069277107 ) ) ;
#4879=EDGE_LOOP ( 'NONE', ( #18763, #9909, #17672, #595 ) ) ;
#4884=ADVANCED_FACE ( 'NONE', ( #20345 ), #246, .T. ) ;
#4887=ORIENTED_EDGE ( 'NONE', *, *, #21733, .F. ) ;
#4894=CARTESIAN_POINT ( 'NONE',  ( 2.915917464538113180, -3.968114999999999615, -18.72348548116188027 ) ) ;
#4895=FACE_OUTER_BOUND ( 'NONE', #15046, .T. ) ;
#4902=DIRECTION ( 'NONE',  ( -0.000000000000000000, -1.000000000000000000, 0.000000000000000000 ) ) ;
#4914=PRODUCT ( 'Ratchet Operating Handle', 'Ratchet Operating Handle', '', ( #19040 ) ) ;
#4918=VECTOR ( 'NONE', #6436, 1000.000000000000000 ) ;
#4922=CARTESIAN_POINT ( 'NONE',  ( 11.75439013559175017, -3.968114999999999615, 4.331204221326972359 ) ) ;
#4929=ORIENTED_EDGE ( 'NONE', *, *, #19106, .T. ) ;
#4930=CARTESIAN_POINT ( 'NONE',  ( 12.02474915109715603, 34.52875999999999834, -13.51434638588835391 ) ) ;
#4932=CARTESIAN_POINT ( 'NONE',  ( 29.45491884992628329, -3.968114999999999615, -15.58809351040512325 ) ) ;
#4952=ORIENTED_EDGE ( 'NONE', *, *, #10578, .T. ) ;
#4965=VECTOR ( 'NONE', #7835, 1000.000000000000000 ) ;
#4966=VECTOR ( 'NONE', #4505, 1000.000000000000000 ) ;
#4969=DIRECTION ( 'NONE',  ( 0.9173788132826626862, 0.000000000000000000, -0.3980152169705242216 ) ) ;
#4971=CARTESIAN_POINT ( 'NONE',  ( 2.915917464538113180, 36.51313500000000545, -18.72348548116188027 ) ) ;
#4977=AXIS2_PLACEMENT_3D ( 'NONE', #136, #2007, #15422 ) ;
#4978=DIRECTION ( 'NONE',  ( -0.9964481331860212121, 0.000000000000000000, 0.08420877549337302259 ) ) ;
#4982=DIRECTION ( 'NONE',  ( 0.2490110332224846346, 0.000000000000000000, -0.9685006480810792739 ) ) ;
#4996=VECTOR ( 'NONE', #8423, 1000.000000000000000 ) ;
#5028=ADVANCED_FACE ( 'NONE', ( #2005 ), #12534, .T. ) ;
#5058=DIRECTION ( 'NONE',  ( 0.000000000000000000, 1.000000000000000000, 0.000000000000000000 ) ) ;
#5060=LINE ( 'NONE', #21858, #11129 ) ;
#5070=VECTOR ( 'NONE', #12144, 1000.000000000000000 ) ;
#5077=ORIENTED_EDGE ( 'NONE', *, *, #7776, .F. ) ;
#5081=CARTESIAN_POINT ( 'NONE',  ( 66.79943102505561114, -1.983739999999999393, -12.07331878313145168 ) ) ;
#5087=FACE_OUTER_BOUND ( 'NONE', #2381, .T. ) ;
#5094=CARTESIAN_POINT ( 'NONE',  ( 11.56192577415882816, 34.52875999999999834, 4.677561850332325299 ) ) ;
#5106=AXIS2_PLACEMENT_3D ( 'NONE', #13338, #13659, #5228 ) ;
#5116=CARTESIAN_POINT ( 'NONE',  ( 10.02683081661366593, -14.84248999999999974, -16.89519978567464165 ) ) ;
#5119=EDGE_LOOP ( 'NONE', ( #3096, #6612, #11662, #3105 ) ) ;
#5122=ORIENTED_EDGE ( 'NONE', *, *, #9518, .T. ) ;
#5131=ORIENTED_EDGE ( 'NONE', *, *, #11855, .F. ) ;
#5154=CARTESIAN_POINT ( 'NONE',  ( 9.256853431388732290, 36.51313500000000545, -17.09316853730597074 ) ) ;
#5155=ORIENTED_EDGE ( 'NONE', *, *, #12493, .T. ) ;
#5156=EDGE_CURVE ( 'NONE', #17362, #6011, #14089, .T. ) ;
#5158=CARTESIAN_POINT ( 'NONE',  ( -16.07247711516169275, 37.85422182005619618, -10.44681224123558039 ) ) ;
#5161=VERTEX_POINT ( 'NONE', #9187 ) ;
#5163=CARTESIAN_POINT ( 'NONE',  ( -16.88621914012359326, -3.266559801243759331, -10.37804376527844141 ) ) ;
#5164=( LENGTH_UNIT ( ) NAMED_UNIT ( * ) SI_UNIT ( .MILLI., .METRE. ) );
#5172=LINE ( 'NONE', #18654, #8527 ) ;
#5174=ADVANCED_FACE ( 'NONE', ( #801 ), #7548, .F. ) ;
#5175=ORIENTED_EDGE ( 'NONE', *, *, #18024, .T. ) ;
#5176=DIRECTION ( 'NONE',  ( 0.000000000000000000, 1.000000000000000000, 0.000000000000000000 ) ) ;
#5183=DIRECTION ( 'NONE',  ( 0.000000000000000000, 1.000000000000000000, 0.000000000000000000 ) ) ;
#5206=CARTESIAN_POINT ( 'NONE',  ( -15.84035234298375094, 34.98745120071231440, -10.46642885967841252 ) ) ;
#5209=CARTESIAN_POINT ( 'NONE',  ( -15.27935546639805331, -3.968114999999999615, -26.04713531390440906 ) ) ;
#5216=VECTOR ( 'NONE', #9245, 1000.000000000000000 ) ;
#5228=DIRECTION ( 'NONE',  ( 0.2490110332224836354, 0.000000000000000000, -0.9685006480810794960 ) ) ;
#5244=DIRECTION ( 'NONE',  ( -0.2490110332224846346, 0.000000000000000000, 0.9685006480810792739 ) ) ;
#5248=ORIENTED_EDGE ( 'NONE', *, *, #10848, .T. ) ;
#5250=FACE_OUTER_BOUND ( 'NONE', #4879, .T. ) ;
#5252=VECTOR ( 'NONE', #13091, 1000.000000000000114 ) ;
#5255=DIRECTION ( 'NONE',  ( -0.9964481331860212121, 0.000000000000000000, 0.08420877549337302259 ) ) ;
#5262=DIRECTION ( 'NONE',  ( -3.089352305546554052E-14, 1.000000000000000000, 2.257689246356112745E-14 ) ) ;
#5264=( NAMED_UNIT ( * ) SI_UNIT ( $, .STERADIAN. ) SOLID_ANGLE_UNIT ( ) );
#5265=AXIS2_PLACEMENT_3D ( 'NONE', #14840, #4442, #7854 ) ;
#5266=DIRECTION ( 'NONE',  ( 0.000000000000000000, 1.000000000000000000, 0.000000000000000000 ) ) ;
#5274=EDGE_LOOP ( 'NONE', ( #11800, #3078, #13265, #12834 ) ) ;
#5291=CYLINDRICAL_SURFACE ( 'NONE', #9940, 9.524999999999996803 ) ;
#5296=ADVANCED_FACE ( 'NONE', ( #2781 ), #13081, .F. ) ;
#5311=CIRCLE ( 'NONE', #8142, 0.7950200000000000600 ) ;
#5312=DIRECTION ( 'NONE',  ( 0.000000000000000000, 1.000000000000000000, 0.000000000000000000 ) ) ;
#5330=ORIENTED_EDGE ( 'NONE', *, *, #14837, .T. ) ;
#5334=VERTEX_POINT ( 'NONE', #11506 ) ;
#5338=DIRECTION ( 'NONE',  ( 0.08420877549337300871, 0.000000000000000000, 0.9964481331860212121 ) ) ;
#5341=VECTOR ( 'NONE', #446, 1000.000000000000114 ) ;
#5342=VECTOR ( 'NONE', #2094, 1000.000000000000114 ) ;
#5344=VERTEX_POINT ( 'NONE', #21344 ) ;
#5349=EDGE_CURVE ( 'NONE', #6418, #2731, #1230, .T. ) ;
#5355=CARTESIAN_POINT ( 'NONE',  ( -15.39353573898878658, 34.79968030885680008, -10.30107656633069979 ) ) ;
#5359=ORIENTED_EDGE ( 'NONE', *, *, #11783, .F. ) ;
#5366=ORIENTED_EDGE ( 'NONE', *, *, #16023, .F. ) ;
#5372=ORIENTED_EDGE ( 'NONE', *, *, #11517, .F. ) ;
#5383=CARTESIAN_POINT ( 'NONE',  ( 46.03750000000000142, -14.84248999999999974, -10.31874999999999964 ) ) ;
#5385=CARTESIAN_POINT ( 'NONE',  ( 44.28293121686854761, -3.968114999999999615, -31.08068102505560759 ) ) ;
#5387=ORIENTED_EDGE ( 'NONE', *, *, #362, .T. ) ;
#5394=VECTOR ( 'NONE', #6395, 1000.000000000000114 ) ;
#5395=EDGE_LOOP ( 'NONE', ( #13484, #6502, #15685, #590 ) ) ;
#5398=VERTEX_POINT ( 'NONE', #5094 ) ;
#5400=DIRECTION ( 'NONE',  ( 0.08420877549337300871, 0.000000000000000000, 0.9964481331860212121 ) ) ;
#5407=LINE ( 'NONE', #445, #1815 ) ;
#5412=VECTOR ( 'NONE', #13798, 1000.000000000000000 ) ;
#5413=DIRECTION ( 'NONE',  ( -0.9685006480810794960, 0.000000000000000000, -0.2490110332224836354 ) ) ;
#5422=VECTOR ( 'NONE', #8181, 1000.000000000000000 ) ;
#5440=DIRECTION ( 'NONE',  ( -0.8741107132214044340, 0.000000000000000000, -0.4857267349359799535 ) ) ;
#5450=FACE_OUTER_BOUND ( 'NONE', #4875, .T. ) ;
#5454=EDGE_CURVE ( 'NONE', #7062, #21627, #2090, .T. ) ;
#5464=CIRCLE ( 'NONE', #12564, 3.970019999999997662 ) ;
#5465=ORIENTED_EDGE ( 'NONE', *, *, #4422, .T. ) ;
#5473=EDGE_CURVE ( 'NONE', #18633, #6373, #15501, .T. ) ;
#5474=ADVANCED_FACE ( 'NONE', ( #7073 ), #5291, .F. ) ;
#5475=CARTESIAN_POINT ( 'NONE',  ( 17.02725982432203367, 34.52875999999999834, -14.27444360421403857 ) ) ;
#5476=EDGE_LOOP ( 'NONE', ( #11894, #17910 ) ) ;
#5479=DIRECTION ( 'NONE',  ( -0.9964481331860212121, 0.000000000000000000, 0.08420877549337336954 ) ) ;
#5483=AXIS2_PLACEMENT_3D ( 'NONE', #10192, #3568, #20451 ) ;
#5497=CARTESIAN_POINT ( 'NONE',  ( 44.28293121686854761, 36.51313500000000545, -31.08068102505560759 ) ) ;
#5514=LINE ( 'NONE', #7295, #11579 ) ;
#5517=CARTESIAN_POINT ( 'NONE',  ( 9.335363283976800375, -3.968114999999999615, -14.20581391854862474 ) ) ;
#5518=CARTESIAN_POINT ( 'NONE',  ( 11.82678039945931481, 34.52875999999999834, -12.74436900065013667 ) ) ;
#5523=CARTESIAN_POINT ( 'NONE',  ( 3.360635606688116894, -14.84248999999999974, -20.45316710734507026 ) ) ;
#5533=CARTESIAN_POINT ( 'NONE',  ( 46.03750000000000142, -1.983739999999999393, -10.31874999999999964 ) ) ;
#5537=CARTESIAN_POINT ( 'NONE',  ( 21.25660046192028929, -1.983739999999999393, -13.18703856829094079 ) ) ;
#5556=LINE ( 'NONE', #7443, #19089 ) ;
#5560=VERTEX_POINT ( 'NONE', #15167 ) ;
#5577=CARTESIAN_POINT ( 'NONE',  ( 11.75439013559175017, -1.983739999999999393, 4.331204221326972359 ) ) ;
#5578=EDGE_CURVE ( 'NONE', #3364, #8815, #552, .T. ) ;
#5583=DIRECTION ( 'NONE',  ( 0.000000000000000000, 1.000000000000000000, 0.000000000000000000 ) ) ;
#5586=LINE ( 'NONE', #12345, #17086 ) ;
#5589=DIRECTION ( 'NONE',  ( -0.08420877549337300871, 0.000000000000000000, -0.9964481331860212121 ) ) ;
#5592=LINE ( 'NONE', #5716, #11038 ) ;
#5597=CIRCLE ( 'NONE', #6655, 1.191259999999999319 ) ;
#5598=VERTEX_POINT ( 'NONE', #15828 ) ;
#5600=DIRECTION ( 'NONE',  ( -0.9964481331860213231, 0.000000000000000000, 0.08420877549337293932 ) ) ;
#5613=EDGE_LOOP ( 'NONE', ( #15507, #18949, #21847, #11900 ) ) ;
#5618=ORIENTED_EDGE ( 'NONE', *, *, #19742, .T. ) ;
#5620=DIRECTION ( 'NONE',  ( 0.08420877549337302259, 0.000000000000000000, 0.9964481331860212121 ) ) ;
#5635=ORIENTED_EDGE ( 'NONE', *, *, #2543, .F. ) ;
#5642=LINE ( 'NONE', #3664, #10236 ) ;
#5651=DIRECTION ( 'NONE',  ( -0.000000000000000000, -1.000000000000000000, 0.000000000000000000 ) ) ;
#5657=CYLINDRICAL_SURFACE ( 'NONE', #6459, 9.524999999999996803 ) ;
#5665=DIRECTION ( 'NONE',  ( 0.000000000000000000, 1.000000000000000000, 0.000000000000000000 ) ) ;
#5675=DIRECTION ( 'NONE',  ( 0.2490110332224846623, 0.000000000000000000, -0.9685006480810793850 ) ) ;
#5689=LINE ( 'NONE', #12560, #6385 ) ;
#5704=CLOSED_SHELL ( 'NONE', ( #5174, #19745, #3025, #8258, #14701, #18661, #9504, #823, #12021, #11364, #8124, #11300, #10854, #10855, #14142, #12280, #17188, #9327, #12372, #20334, #1779, #2103, #16522, #7803, #20562, #17570, #13980, #5296, #3968, #3277, #10029, #18041, #899, #15115, #13762, #19133, #4019, #18292, #556, #12076, #6490, #4664, #5028, #12566, #4821, #12235, #11974, #211, #9747, #8298, #16237, #16302, #3745, #8203, #6531, #19926, #13876, #2160, #13715, #20591, #7500, #4865, #11397, #13095, #20936, #5474, #10331, #898, #3698, #10903, #1517, #519, #18676, #12629, #15157, #1431, #10175, #16801, #16824, #10779, #21397, #8714, #15213, #9942, #17520, #15183, #451, #11575, #2886, #11554, #4884, #88, #618, #2473, #15888, #1377 ) ) ;
#5706=ORIENTED_EDGE ( 'NONE', *, *, #4378, .F. ) ;
#5709=VECTOR ( 'NONE', #17025, 1000.000000000000000 ) ;
#5714=EDGE_CURVE ( 'NONE', #9371, #2216, #17689, .T. ) ;
#5715=EDGE_CURVE ( 'NONE', #11228, #9683, #3986, .T. ) ;
#5716=CARTESIAN_POINT ( 'NONE',  ( 19.79515554403045741, -3.968114999999999615, -10.69562145279641996 ) ) ;
#5717=AXIS2_PLACEMENT_3D ( 'NONE', #545, #17680, #15600 ) ;
#5722=CARTESIAN_POINT ( 'NONE',  ( -16.73439918454169018, 37.15413452960619622, -25.92417111164088084 ) ) ;
#5723=CARTESIAN_POINT ( 'NONE',  ( -21.45091887247874851, 40.79338547039380103, -9.992285829511605044 ) ) ;
#5725=DIRECTION ( 'NONE',  ( -0.08420877549337300871, 0.000000000000000000, -0.9964481331860212121 ) ) ;
#5728=AXIS2_PLACEMENT_3D ( 'NONE', #12713, #19438, #11050 ) ;
#5740=VECTOR ( 'NONE', #8220, 1000.000000000000114 ) ;
#5741=CIRCLE ( 'NONE', #19498, 1.785937499999998179 ) ;
#5747=ORIENTED_EDGE ( 'NONE', *, *, #21637, .F. ) ;
#5756=FACE_OUTER_BOUND ( 'NONE', #19984, .T. ) ;
#5765=EDGE_CURVE ( 'NONE', #1238, #2549, #6281, .T. ) ;
#5769=DIRECTION ( 'NONE',  ( -0.000000000000000000, -1.000000000000000000, 0.000000000000000000 ) ) ;
#5781=DIRECTION ( 'NONE',  ( 0.2490110332224836354, 0.000000000000000000, -0.9685006480810794960 ) ) ;
#5783=ORIENTED_EDGE ( 'NONE', *, *, #1953, .F. ) ;
#5784=VECTOR ( 'NONE', #13500, 1000.000000000000114 ) ;
#5785=CARTESIAN_POINT ( 'NONE',  ( 3.805353748838121053, -14.84248999999999974, -22.18284873352824960 ) ) ;
#5790=ORIENTED_EDGE ( 'NONE', *, *, #14371, .T. ) ;
#5798=VECTOR ( 'NONE', #17681, 1000.000000000000114 ) ;
#5822=ORIENTED_EDGE ( 'NONE', *, *, #6411, .F. ) ;
#5825=AXIS2_PLACEMENT_3D ( 'NONE', #11835, #6853, #17136 ) ;
#5827=ORIENTED_EDGE ( 'NONE', *, *, #21445, .F. ) ;
#5830=ORIENTED_EDGE ( 'NONE', *, *, #10058, .T. ) ;
#5833=VERTEX_POINT ( 'NONE', #19760 ) ;
#5843=DIRECTION ( 'NONE',  ( 0.000000000000000000, 1.000000000000000000, 0.000000000000000000 ) ) ;
#5847=DIRECTION ( 'NONE',  ( -0.000000000000000000, -1.000000000000000000, 0.000000000000000000 ) ) ;
#5874=DIRECTION ( 'NONE',  ( -0.9964481331860213231, 0.000000000000000000, 0.08420877549337293932 ) ) ;
#5877=ORIENTED_EDGE ( 'NONE', *, *, #18022, .T. ) ;
#5879=DIRECTION ( 'NONE',  ( 0.000000000000000000, -1.000000000000000000, 0.000000000000000000 ) ) ;
#5890=DIRECTION ( 'NONE',  ( 0.000000000000000000, 1.000000000000000000, 0.000000000000000000 ) ) ;
#5891=ORIENTED_EDGE ( 'NONE', *, *, #674, .T. ) ;
#5918=ORIENTED_EDGE ( 'NONE', *, *, #16412, .T. ) ;
#5925=DIRECTION ( 'NONE',  ( 0.2490110332224836354, 0.000000000000000000, -0.9685006480810794960 ) ) ;
#5928=ORIENTED_EDGE ( 'NONE', *, *, #13438, .F. ) ;
#5934=VERTEX_POINT ( 'NONE', #15371 ) ;
#5939=MANIFOLD_SOLID_BREP ( 'Stock-MAS-676-1', #5704 ) ;
#5940=DIRECTION ( 'NONE',  ( 0.7334850928793767988, -0.6768732144311027099, -0.06198604769976990420 ) ) ;
#5945=EDGE_CURVE ( 'NONE', #7624, #8950, #14929, .T. ) ;
#5955=CARTESIAN_POINT ( 'NONE',  ( -16.07247711516169275, 35.13319853559599437, -10.44681224123558039 ) ) ;
#5959=VERTEX_POINT ( 'NONE', #18644 ) ;
#5961=AXIS2_PLACEMENT_3D ( 'NONE', #1309, #18232, #19983 ) ;
#5975=CARTESIAN_POINT ( 'NONE',  ( 11.75439013559175017, 128.5105379999999968, 4.331204221326972359 ) ) ;
#5981=DIRECTION ( 'NONE',  ( 0.000000000000000000, 1.000000000000000000, 0.000000000000000000 ) ) ;
#5999=VECTOR ( 'NONE', #15219, 1000.000000000000114 ) ;
#6004=EDGE_CURVE ( 'NONE', #337, #8462, #12146, .T. ) ;
#6005=EDGE_CURVE ( 'NONE', #11084, #14947, #7484, .T. ) ;
#6011=VERTEX_POINT ( 'NONE', #848 ) ;
#6012=FACE_OUTER_BOUND ( 'NONE', #8228, .T. ) ;
#6020=ORIENTED_EDGE ( 'NONE', *, *, #882, .T. ) ;
#6037=ORIENTED_EDGE ( 'NONE', *, *, #6004, .F. ) ;
#6038=DIRECTION ( 'NONE',  ( 0.9636276526537417286, 0.000000000000000000, -0.2672484743474499158 ) ) ;
#6040=ORIENTED_EDGE ( 'NONE', *, *, #437, .T. ) ;
#6051=VECTOR ( 'NONE', #16500, 1000.000000000000000 ) ;
#6059=CARTESIAN_POINT ( 'NONE',  ( -46.55710204590916135, -8.889364999999999739, -7.870588902259476605 ) ) ;
#6063=VERTEX_POINT ( 'NONE', #20049 ) ;
#6069=ORIENTED_EDGE ( 'NONE', *, *, #14771, .T. ) ;
#6104=FACE_OUTER_BOUND ( 'NONE', #13488, .T. ) ;
#6113=CIRCLE ( 'NONE', #21664, 15.47812499999999680 ) ;
#6122=LINE ( 'NONE', #13324, #20122 ) ;
#6124=CARTESIAN_POINT ( 'NONE',  ( 17.79723720954694954, -1.983739999999999393, -14.07647485258271303 ) ) ;
#6125=EDGE_CURVE ( 'NONE', #10206, #20031, #15597, .T. ) ;
#6126=CARTESIAN_POINT ( 'NONE',  ( -47.86112874365709047, -5.714999999999999858, -23.29368419115692035 ) ) ;
#6129=DIRECTION ( 'NONE',  ( 0.2490110332224857170, 0.000000000000000000, -0.9685006480810790519 ) ) ;
#6147=DIRECTION ( 'NONE',  ( -0.9685006480810792739, 0.000000000000000000, -0.2490110332224846346 ) ) ;
#6157=ORIENTED_EDGE ( 'NONE', *, *, #11852, .T. ) ;
#6163=DIRECTION ( 'NONE',  ( -0.9964481331860212121, 0.000000000000000000, 0.08420877549337303647 ) ) ;
#6172=CARTESIAN_POINT ( 'NONE',  ( 12.59675778470975516, -14.84248999999999974, -12.54640024901842033 ) ) ;
#6182=VERTEX_POINT ( 'NONE', #21832 ) ;
#6186=DIRECTION ( 'NONE',  ( 0.2490110332224846623, 0.000000000000000000, -0.9685006480810793850 ) ) ;
#6191=ORIENTED_EDGE ( 'NONE', *, *, #12203, .T. ) ;
#6217=DIRECTION ( 'NONE',  ( -0.000000000000000000, -1.000000000000000000, 0.000000000000000000 ) ) ;
#6232=DIRECTION ( 'NONE',  ( 0.9685006480810790519, 0.000000000000000000, 0.2490110332224857170 ) ) ;
#6239=EDGE_LOOP ( 'NONE', ( #18212, #12455, #9928, #6494 ) ) ;
#6242=DIRECTION ( 'NONE',  ( 0.000000000000000000, 1.000000000000000000, 0.000000000000000000 ) ) ;
#6243=ORIENTED_EDGE ( 'NONE', *, *, #149, .F. ) ;
#6246=ORIENTED_EDGE ( 'NONE', *, *, #15458, .T. ) ;
#6253=EDGE_CURVE ( 'NONE', #9783, #8950, #18714, .T. ) ;
#6254=ORIENTED_EDGE ( 'NONE', *, *, #5578, .F. ) ;
#6259=VERTEX_POINT ( 'NONE', #10322 ) ;
#6266=ORIENTED_EDGE ( 'NONE', *, *, #18200, .F. ) ;
#6267=CIRCLE ( 'NONE', #1667, 0.7950200000000000600 ) ;
#6268=ORIENTED_EDGE ( 'NONE', *, *, #2393, .F. ) ;
#6271=EDGE_CURVE ( 'NONE', #21107, #5161, #1692, .T. ) ;
#6278=EDGE_CURVE ( 'NONE', #11569, #19768, #10299, .T. ) ;
#6281=LINE ( 'NONE', #1205, #4965 ) ;
#6282=DIRECTION ( 'NONE',  ( 0.08420877549337302259, 0.000000000000000000, 0.9964481331860212121 ) ) ;
#6296=CARTESIAN_POINT ( 'NONE',  ( 31.83819605565793509, -3.968114999999999615, -4.158220719828246814 ) ) ;
#6320=DIRECTION ( 'NONE',  ( -0.2672484743474505819, 0.000000000000000000, -0.9636276526537416176 ) ) ;
#6321=DIRECTION ( 'NONE',  ( -0.000000000000000000, -1.000000000000000000, 0.000000000000000000 ) ) ;
#6323=VECTOR ( 'NONE', #10556, 1000.000000000000000 ) ;
#6326=LINE ( 'NONE', #16418, #18686 ) ;
#6341=CARTESIAN_POINT ( 'NONE',  ( 22.02657784715807665, -3.968114999999999615, -12.98906981665815330 ) ) ;
#6346=ORIENTED_EDGE ( 'NONE', *, *, #6413, .T. ) ;
#6347=CARTESIAN_POINT ( 'NONE',  ( 28.56548256563643662, -3.968114999999999615, -12.12873025803960658 ) ) ;
#6364=CIRCLE ( 'NONE', #6713, 0.7950200000000000600 ) ;
#6365=DIRECTION ( 'NONE',  ( -0.000000000000000000, -1.000000000000000000, 0.000000000000000000 ) ) ;
#6367=DIRECTION ( 'NONE',  ( -0.9685006480810793850, 0.000000000000000000, -0.2490110332224846623 ) ) ;
#6373=VERTEX_POINT ( 'NONE', #18391 ) ;
#6382=CARTESIAN_POINT ( 'NONE',  ( -47.86112874365709047, -10.87373999999999974, -23.29368419115692035 ) ) ;
#6385=VECTOR ( 'NONE', #932, 1000.000000000000000 ) ;
#6392=VECTOR ( 'NONE', #14910, 1000.000000000000000 ) ;
#6395=DIRECTION ( 'NONE',  ( -0.9685006480810792739, 0.000000000000000000, -0.2490110332224846346 ) ) ;
#6404=EDGE_CURVE ( 'NONE', #14366, #7791, #20497, .T. ) ;
#6411=EDGE_CURVE ( 'NONE', #9888, #21307, #13828, .T. ) ;
#6413=EDGE_CURVE ( 'NONE', #1375, #5344, #8874, .T. ) ;
#6414=CARTESIAN_POINT ( 'NONE',  ( -15.40791870427606369, 37.14670541160712958, -10.30897195908432451 ) ) ;
#6418=VERTEX_POINT ( 'NONE', #7240 ) ;
#6424=CIRCLE ( 'NONE', #15637, 0.7950200000000000600 ) ;
#6425=ORIENTED_EDGE ( 'NONE', *, *, #967, .F. ) ;
#6430=VERTEX_POINT ( 'NONE', #20469 ) ;
#6436=DIRECTION ( 'NONE',  ( -0.000000000000000000, -1.000000000000000000, 0.000000000000000000 ) ) ;
#6455=ORIENTED_EDGE ( 'NONE', *, *, #10218, .T. ) ;
#6459=AXIS2_PLACEMENT_3D ( 'NONE', #11079, #14199, #579 ) ;
#6483=AXIS2_PLACEMENT_3D ( 'NONE', #236, #13744, #5312 ) ;
#6488=ORIENTED_EDGE ( 'NONE', *, *, #11943, .F. ) ;
#6489=ORIENTED_EDGE ( 'NONE', *, *, #37, .T. ) ;
#6490=ADVANCED_FACE ( 'NONE', ( #15869 ), #20807, .T. ) ;
#6494=ORIENTED_EDGE ( 'NONE', *, *, #14416, .F. ) ;
#6499=EDGE_CURVE ( 'NONE', #21254, #14428, #5556, .T. ) ;
#6500=( BOUNDED_CURVE ( )  B_SPLINE_CURVE ( 3, ( #6663, #13425, #13540, #9989 ),
 .UNSPECIFIED., .F., .T. ) 
 B_SPLINE_CURVE_WITH_KNOTS ( ( 4, 4 ),
 ( 0.9998823759999307947, 1.570796326793153508 ),
 .UNSPECIFIED. ) 
 CURVE ( )  GEOMETRIC_REPRESENTATION_ITEM ( )  RATIONAL_B_SPLINE_CURVE ( ( 1.000000000000000000, 0.9730220469484401891, 0.9730220469484401891, 1.000000000000000000 ) ) 
 REPRESENTATION_ITEM ( '' )  );
#6502=ORIENTED_EDGE ( 'NONE', *, *, #16836, .T. ) ;
#6507=AXIS2_PLACEMENT_3D ( 'NONE', #19172, #4252, #19051 ) ;
#6513=CARTESIAN_POINT ( 'NONE',  ( 56.47666780297049627, 34.52875999999999834, 1.109116340531466127 ) ) ;
#6516=FACE_OUTER_BOUND ( 'NONE', #15537, .T. ) ;
#6517=ORIENTED_EDGE ( 'NONE', *, *, #17057, .F. ) ;
#6530=CARTESIAN_POINT ( 'NONE',  ( -53.00154558624916490, -10.87373999999999974, -22.85927301266823264 ) ) ;
#6531=ADVANCED_FACE ( 'NONE', ( #4354 ), #11196, .F. ) ;
#6535=CYLINDRICAL_SURFACE ( 'NONE', #15130, 5.158739999999997217 ) ;
#6541=ORIENTED_EDGE ( 'NONE', *, *, #17264, .F. ) ;
#6551=DIRECTION ( 'NONE',  ( -0.9636276526537417286, 0.000000000000000000, 0.2672484743474501934 ) ) ;
#6554=DIRECTION ( 'NONE',  ( 0.08420877549337300871, 0.000000000000000000, 0.9964481331860212121 ) ) ;
#6558=CARTESIAN_POINT ( 'NONE',  ( 28.56548256563643662, 34.52875999999999834, -12.12873025803960658 ) ) ;
#6560=DIRECTION ( 'NONE',  ( 0.000000000000000000, 1.000000000000000000, 0.000000000000000000 ) ) ;
#6579=ORIENTED_EDGE ( 'NONE', *, *, #14771, .F. ) ;
#6591=CARTESIAN_POINT ( 'NONE',  ( -22.90596259062238005, 39.45064500000000152, -9.869321627248080375 ) ) ;
#6600=EDGE_LOOP ( 'NONE', ( #12483, #15620, #18280, #14881 ) ) ;
#6612=ORIENTED_EDGE ( 'NONE', *, *, #6004, .T. ) ;
#6613=VERTEX_POINT ( 'NONE', #19694 ) ;
#6616=VERTEX_POINT ( 'NONE', #4564 ) ;
#6630=DIRECTION ( 'NONE',  ( -0.000000000000000000, -1.000000000000000000, 0.000000000000000000 ) ) ;
#6633=EDGE_LOOP ( 'NONE', ( #7330, #14847, #21362, #17102, #458, #19988, #9054, #11106, #5248, #18635, #11826, #14362, #14352, #14492, #16802, #9448, #9344, #15406, #13002, #17947, #20029 ) ) ;
#6638=ORIENTED_EDGE ( 'NONE', *, *, #17505, .T. ) ;
#6652=CARTESIAN_POINT ( 'NONE',  ( -15.39353573898878658, -4.587157632697119958, -10.30107656633069979 ) ) ;
#6655=AXIS2_PLACEMENT_3D ( 'NONE', #19397, #4271, #9343 ) ;
#6660=ORIENTED_EDGE ( 'NONE', *, *, #17146, .F. ) ;
#6663=CARTESIAN_POINT ( 'NONE',  ( -15.41509608936259035, -4.609114529603660415, -10.31276839742836415 ) ) ;
#6667=CARTESIAN_POINT ( 'NONE',  ( -51.69815163306579819, -5.714999999999999858, -7.436124251198355850 ) ) ;
#6679=VECTOR ( 'NONE', #2491, 1000.000000000000114 ) ;
#6681=EDGE_LOOP ( 'NONE', ( #4075, #2413, #15806, #5465 ) ) ;
#6694=ORIENTED_EDGE ( 'NONE', *, *, #13364, .F. ) ;
#6698=CIRCLE ( 'NONE', #19750, 1.191259999999999319 ) ;
#6701=VERTEX_POINT ( 'NONE', #19916 ) ;
#6707=ORIENTED_EDGE ( 'NONE', *, *, #2393, .T. ) ;
#6713=AXIS2_PLACEMENT_3D ( 'NONE', #13644, #3361, #20240 ) ;
#6714=CARTESIAN_POINT ( 'NONE',  ( -51.02421882195815783, 41.43438499999999891, -23.02637480153789795 ) ) ;
#6717=DIRECTION ( 'NONE',  ( 0.08420877549337300871, 0.000000000000000000, 0.9964481331860212121 ) ) ;
#6720=CARTESIAN_POINT ( 'NONE',  ( 9.828862065001116477, 36.51313500000000545, -16.12522240043857025 ) ) ;
#6723=ORIENTED_EDGE ( 'NONE', *, *, #2518, .T. ) ;
#6727=ORIENTED_EDGE ( 'NONE', *, *, #16187, .F. ) ;
#6728=VERTEX_POINT ( 'NONE', #8309 ) ;
#6731=VERTEX_POINT ( 'NONE', #21578 ) ;
#6732=CIRCLE ( 'NONE', #19079, 3.174999999999999378 ) ;
#6740=CARTESIAN_POINT ( 'NONE',  ( 19.79515554403045741, 36.51313500000000545, -10.69562145279641996 ) ) ;
#6741=ORIENTED_EDGE ( 'NONE', *, *, #8716, .F. ) ;
#6744=CARTESIAN_POINT ( 'NONE',  ( 9.256853431388732290, 34.52875999999999834, -17.09316853730597074 ) ) ;
#6746=VECTOR ( 'NONE', #7108, 1000.000000000000000 ) ;
#6752=AXIS2_PLACEMENT_3D ( 'NONE', #2467, #7435, #7112 ) ;
#6753=EDGE_CURVE ( 'NONE', #5934, #10166, #7783, .T. ) ;
#6760=CIRCLE ( 'NONE', #10652, 1.191259999999999097 ) ;
#6785=ORIENTED_EDGE ( 'NONE', *, *, #16533, .T. ) ;
#6788=VECTOR ( 'NONE', #9129, 1000.000000000000114 ) ;
#6789=DIRECTION ( 'NONE',  ( 0.000000000000000000, 1.000000000000000000, 0.000000000000000000 ) ) ;
#6793=CIRCLE ( 'NONE', #11744, 3.174999999999998934 ) ;
#6799=EDGE_CURVE ( 'NONE', #19334, #14145, #15011, .T. ) ;
#6802=CARTESIAN_POINT ( 'NONE',  ( 9.256853431388732290, -3.968114999999999615, -17.09316853730597074 ) ) ;
#6816=CYLINDRICAL_SURFACE ( 'NONE', #21827, 1.983739999999999393 ) ;
#6824=CARTESIAN_POINT ( 'NONE',  ( 30.42699695299585017, -3.968114999999999615, -4.832012189960551041 ) ) ;
#6830=EDGE_CURVE ( 'NONE', #10784, #6991, #13971, .T. ) ;
#6836=DIRECTION ( 'NONE',  ( 0.9964481331860212121, 0.000000000000000000, -0.08420877549337300871 ) ) ;
#6844=ORIENTED_EDGE ( 'NONE', *, *, #9397, .F. ) ;
#6849=DIRECTION ( 'NONE',  ( 0.000000000000000000, 1.000000000000000000, 0.000000000000000000 ) ) ;
#6850=CIRCLE ( 'NONE', #10373, 9.525000000000002132 ) ;
#6853=DIRECTION ( 'NONE',  ( 0.000000000000000000, 1.000000000000000000, 0.000000000000000000 ) ) ;
#6856=LINE ( 'NONE', #6740, #9455 ) ;
#6862=CARTESIAN_POINT ( 'NONE',  ( 12.25799425556778388, -3.968114999999999615, 0.2069032437451798767 ) ) ;
#6863=DIRECTION ( 'NONE',  ( -0.2490110332224846346, 0.000000000000000000, 0.9685006480810792739 ) ) ;
#6866=DIRECTION ( 'NONE',  ( -0.9964481331860209901, 0.000000000000000000, 0.08420877549337456303 ) ) ;
#6868=EDGE_LOOP ( 'NONE', ( #13462, #5747, #12101, #10674 ) ) ;
#6869=CIRCLE ( 'NONE', #3010, 15.47812499999999680 ) ;
#6881=DIRECTION ( 'NONE',  ( 0.08420877549337300871, 0.000000000000000000, 0.9964481331860212121 ) ) ;
#6884=DIRECTION ( 'NONE',  ( 0.000000000000000000, 1.000000000000000000, 0.000000000000000000 ) ) ;
#6888=CARTESIAN_POINT ( 'NONE',  ( 22.22454659879084460, -1.983739999999999393, -13.75904720189594244 ) ) ;
#6889=ORIENTED_EDGE ( 'NONE', *, *, #17854, .T. ) ;
#6905=CARTESIAN_POINT ( 'NONE',  ( 36.54633153140314761, 34.52875999999999834, -9.516661413425623550 ) ) ;
#6926=EDGE_CURVE ( 'NONE', #374, #19312, #666, .T. ) ;
#6927=EDGE_CURVE ( 'NONE', #1, #10166, #5642, .T. ) ;
#6937=DIRECTION ( 'NONE',  ( 0.2490110332224848289, 0.000000000000000000, -0.9685006480810792739 ) ) ;
#6939=VERTEX_POINT ( 'NONE', #20327 ) ;
#6943=CARTESIAN_POINT ( 'NONE',  ( 17.22522857595987844, 36.51313500000000545, -15.04442098945225403 ) ) ;
#6945=ORIENTED_EDGE ( 'NONE', *, *, #336, .T. ) ;
#6946=CARTESIAN_POINT ( 'NONE',  ( -51.69815163306579819, 38.26001999999999725, -7.436124251198355850 ) ) ;
#6948=ORIENTED_EDGE ( 'NONE', *, *, #14837, .F. ) ;
#6953=CARTESIAN_POINT ( 'NONE',  ( 11.75439013559175017, 34.52875999999999834, 4.331204221326972359 ) ) ;
#6955=FACE_OUTER_BOUND ( 'NONE', #8872, .T. ) ;
#6968=VERTEX_POINT ( 'NONE', #2766 ) ;
#6969=CARTESIAN_POINT ( 'NONE',  ( 3.805353748838121053, 36.51313500000000545, -22.18284873352824960 ) ) ;
#6977=LINE ( 'NONE', #20335, #12171 ) ;
#6978=CARTESIAN_POINT ( 'NONE',  ( -22.75431282566211522, -8.248365470396340271, -25.41543459098148716 ) ) ;
#6991=VERTEX_POINT ( 'NONE', #4208 ) ;
#6993=LINE ( 'NONE', #11874, #3138 ) ;
#7001=CARTESIAN_POINT ( 'NONE',  ( -16.07247711516169275, -5.309201820043501385, -10.44681224123558039 ) ) ;
#7003=VECTOR ( 'NONE', #11618, 1000.000000000000000 ) ;
#7004=ORIENTED_EDGE ( 'NONE', *, *, #20453, .T. ) ;
#7016=ORIENTED_EDGE ( 'NONE', *, *, #11524, .T. ) ;
#7019=CARTESIAN_POINT ( 'NONE',  ( -47.86049599909252805, -8.889364999999999739, -23.29373766372935961 ) ) ;
#7027=ORIENTED_EDGE ( 'NONE', *, *, #21796, .F. ) ;
#7034=CARTESIAN_POINT ( 'NONE',  ( 20.76310168089343478, 34.52875999999999834, -11.26763008640078212 ) ) ;
#7043=CARTESIAN_POINT ( 'NONE',  ( 18.07371581377308800, 34.52875999999999834, -11.95909761906105473 ) ) ;
#7051=DIRECTION ( 'NONE',  ( -0.08420877549337300871, 0.000000000000000000, -0.9964481331860212121 ) ) ;
#7054=ORIENTED_EDGE ( 'NONE', *, *, #8671, .F. ) ;
#7057=AXIS2_PLACEMENT_3D ( 'NONE', #1800, #10102, #11876 ) ;
#7062=VERTEX_POINT ( 'NONE', #988 ) ;
#7068=DIRECTION ( 'NONE',  ( 0.2490110332224857170, 0.000000000000000000, -0.9685006480810790519 ) ) ;
#7069=AXIS2_PLACEMENT_3D ( 'NONE', #20332, #15080, #11518 ) ;
#7070=VERTEX_POINT ( 'NONE', #19450 ) ;
#7073=FACE_OUTER_BOUND ( 'NONE', #4841, .T. ) ;
#7075=DIRECTION ( 'NONE',  ( -0.2490110332224848011, 0.000000000000000000, 0.9685006480810792739 ) ) ;
#7076=ORIENTED_EDGE ( 'NONE', *, *, #12544, .T. ) ;
#7079=FACE_OUTER_BOUND ( 'NONE', #15007, .T. ) ;
#7088=EDGE_CURVE ( 'NONE', #10693, #2731, #10842, .T. ) ;
#7093=CARTESIAN_POINT ( 'NONE',  ( 30.42699695299585017, -3.968114999999999615, -4.832012189960551041 ) ) ;
#7108=DIRECTION ( 'NONE',  ( 0.9636276526537417286, 0.000000000000000000, -0.2672484743474500268 ) ) ;
#7109=CIRCLE ( 'NONE', #13829, 1.983739999999997838 ) ;
#7112=DIRECTION ( 'NONE',  ( 0.4857267349359797870, 0.000000000000000000, -0.8741107132214044340 ) ) ;
#7126=ORIENTED_EDGE ( 'NONE', *, *, #2516, .F. ) ;
#7138=ORIENTED_EDGE ( 'NONE', *, *, #17673, .F. ) ;
#7146=LINE ( 'NONE', #13912, #3976 ) ;
#7149=ORIENTED_EDGE ( 'NONE', *, *, #15032, .T. ) ;
#7152=DIRECTION ( 'NONE',  ( -0.9685006480810792739, 0.000000000000000000, -0.2490110332224846346 ) ) ;
#7155=DIRECTION ( 'NONE',  ( -0.000000000000000000, -1.000000000000000000, 0.000000000000000000 ) ) ;
#7168=DIRECTION ( 'NONE',  ( -0.2490110332224846346, 0.000000000000000000, 0.9685006480810792739 ) ) ;
#7176=VERTEX_POINT ( 'NONE', #11828 ) ;
#7187=CARTESIAN_POINT ( 'NONE',  ( 1.581041518826207248, 34.52875999999999834, -20.30277549736237575 ) ) ;
#7188=AXIS2_PLACEMENT_3D ( 'NONE', #9244, #16027, #6038 ) ;
#7191=LINE ( 'NONE', #649, #8629 ) ;
#7201=ORIENTED_EDGE ( 'NONE', *, *, #2950, .T. ) ;
#7240=CARTESIAN_POINT ( 'NONE',  ( 11.42842559562532578, 34.52875999999999834, 1.673196738795719174 ) ) ;
#7241=FACE_OUTER_BOUND ( 'NONE', #16232, .T. ) ;
#7250=DIRECTION ( 'NONE',  ( -0.2490110332224836354, 0.000000000000000000, 0.9685006480810794960 ) ) ;
#7251=ORIENTED_EDGE ( 'NONE', *, *, #19539, .F. ) ;
#7254=CYLINDRICAL_SURFACE ( 'NONE', #8089, 0.7950200000000000600 ) ;
#7258=CARTESIAN_POINT ( 'NONE',  ( -15.27935546639805331, 38.49687500000000284, -26.04713531390440906 ) ) ;
#7270=PLANE ( 'NONE',  #3278 ) ;
#7275=CARTESIAN_POINT ( 'NONE',  ( -15.39353573898878658, 34.79968030885680008, -10.30107656633069979 ) ) ;
#7295=CARTESIAN_POINT ( 'NONE',  ( -13.87568970999206108, -1.983739999999999393, -9.457638332870221376 ) ) ;
#7300=CYLINDRICAL_SURFACE ( 'NONE', #7831, 9.524999999999996803 ) ;
#7302=EDGE_LOOP ( 'NONE', ( #11056, #12267, #9229, #11291 ) ) ;
#7316=DIRECTION ( 'NONE',  ( 0.08420877549337300871, 0.000000000000000000, 0.9964481331860212121 ) ) ;
#7317=CARTESIAN_POINT ( 'NONE',  ( 14.05820270259704152, 128.5105379999999968, -15.03781736451272444 ) ) ;
#7330=ORIENTED_EDGE ( 'NONE', *, *, #212, .T. ) ;
#7375=DIRECTION ( 'NONE',  ( 0.000000000000000000, 1.000000000000000000, 0.000000000000000000 ) ) ;
#7410=ORIENTED_EDGE ( 'NONE', *, *, #15903, .F. ) ;
#7411=ORIENTED_EDGE ( 'NONE', *, *, #21537, .T. ) ;
#7420=VECTOR ( 'NONE', #18794, 1000.000000000000000 ) ;
#7425=CARTESIAN_POINT ( 'NONE',  ( 44.28293121686854761, 34.52875999999999834, -31.08068102505560759 ) ) ;
#7431=DIRECTION ( 'NONE',  ( -0.000000000000000000, -1.000000000000000000, 0.000000000000000000 ) ) ;
#7435=DIRECTION ( 'NONE',  ( 0.000000000000000000, 1.000000000000000000, 0.000000000000000000 ) ) ;
#7439=CARTESIAN_POINT ( 'NONE',  ( -53.00154558624916490, -5.714999999999999858, -22.85927301266823264 ) ) ;
#7443=CARTESIAN_POINT ( 'NONE',  ( 21.25660046192028929, -1.983739999999999393, -13.18703856829094079 ) ) ;
#7461=EDGE_CURVE ( 'NONE', #1622, #21739, #3639, .T. ) ;
#7467=CARTESIAN_POINT ( 'NONE',  ( 9.335363283976800375, 34.52875999999999834, -14.20581391854862474 ) ) ;
#7474=PLANE ( 'NONE',  #3476 ) ;
#7484=LINE ( 'NONE', #17657, #11737 ) ;
#7487=( GEOMETRIC_REPRESENTATION_CONTEXT ( 3 ) GLOBAL_UNCERTAINTY_ASSIGNED_CONTEXT ( ( #3929 ) ) GLOBAL_UNIT_ASSIGNED_CONTEXT ( ( #5164, #193, #5264 ) ) REPRESENTATION_CONTEXT ( 'NONE', 'WORKASPACE' ) );
#7493=DIRECTION ( 'NONE',  ( -0.000000000000000000, -1.000000000000000000, 0.000000000000000000 ) ) ;
#7500=ADVANCED_FACE ( 'NONE', ( #17009 ), #725, .T. ) ;
#7508=CIRCLE ( 'NONE', #20920, 0.7950200000000000600 ) ;
#7528=ORIENTED_EDGE ( 'NONE', *, *, #15943, .F. ) ;
#7538=AXIS2_PLACEMENT_3D ( 'NONE', #2177, #8919, #298 ) ;
#7548=CYLINDRICAL_SURFACE ( 'NONE', #755, 9.524999999999996803 ) ;
#7551=CARTESIAN_POINT ( 'NONE',  ( 3.360635606688116894, 34.52875999999999834, -20.45316710734507026 ) ) ;
#7576=DIRECTION ( 'NONE',  ( 0.000000000000000000, 1.000000000000000000, 0.000000000000000000 ) ) ;
#7579=DIRECTION ( 'NONE',  ( -0.9173788132826627972, 0.000000000000000000, 0.3980152169705239440 ) ) ;
#7582=DIRECTION ( 'NONE',  ( -0.08420877549337300871, 0.000000000000000000, -0.9964481331860212121 ) ) ;
#7604=DIRECTION ( 'NONE',  ( 0.08420877549337300871, 0.000000000000000000, 0.9964481331860212121 ) ) ;
#7612=ORIENTED_EDGE ( 'NONE', *, *, #13734, .T. ) ;
#7615=DIRECTION ( 'NONE',  ( -0.08420877549337300871, 0.000000000000000000, -0.9964481331860212121 ) ) ;
#7616=CARTESIAN_POINT ( 'NONE',  ( 66.79943102505561114, 34.52875999999999834, -12.07331878313145168 ) ) ;
#7617=DIRECTION ( 'NONE',  ( -0.6744690509234928522, -0.7360996206939028896, 0.05699866455150636585 ) ) ;
#7618=CARTESIAN_POINT ( 'NONE',  ( 17.79723720954694954, -1.983739999999999393, -14.07647485258271303 ) ) ;
#7622=CARTESIAN_POINT ( 'NONE',  ( 9.256853431388732290, -1.983739999999999393, -17.09316853730597074 ) ) ;
#7624=VERTEX_POINT ( 'NONE', #6347 ) ;
#7625=ORIENTED_EDGE ( 'NONE', *, *, #16956, .F. ) ;
#7627=LINE ( 'NONE', #12843, #950 ) ;
#7637=DIRECTION ( 'NONE',  ( 0.08420877549337300871, 0.000000000000000000, 0.9964481331860212121 ) ) ;
#7644=LINE ( 'NONE', #16386, #12704 ) ;
#7647=FACE_OUTER_BOUND ( 'NONE', #15764, .T. ) ;
#7655=ORIENTED_EDGE ( 'NONE', *, *, #11833, .F. ) ;
#7665=CIRCLE ( 'NONE', #14389, 0.7950200000000003930 ) ;
#7677=ORIENTED_EDGE ( 'NONE', *, *, #14838, .T. ) ;
#7680=CYLINDRICAL_SURFACE ( 'NONE', #3503, 3.174999999999997158 ) ;
#7684=LINE ( 'NONE', #21485, #17649 ) ;
#7719=CARTESIAN_POINT ( 'NONE',  ( -19.26602273594821924, 38.49687500000000284, -73.22163862549463431 ) ) ;
#7722=DIRECTION ( 'NONE',  ( 0.000000000000000000, 1.000000000000000000, 0.000000000000000000 ) ) ;
#7725=DIRECTION ( 'NONE',  ( 0.9964481331860212121, 0.000000000000000000, -0.08420877549337300871 ) ) ;
#7727=DIRECTION ( 'NONE',  ( -0.9685006480810792739, 0.000000000000000000, -0.2490110332224846346 ) ) ;
#7749=FACE_BOUND ( 'NONE', #11573, .T. ) ;
#7771=CARTESIAN_POINT ( 'NONE',  ( 21.45456921355305724, -14.84248999999999974, -13.95701595352872815 ) ) ;
#7776=EDGE_CURVE ( 'NONE', #3833, #7070, #19850, .T. ) ;
#7777=CARTESIAN_POINT ( 'NONE',  ( -15.27935546639805331, -5.951855000000001006, -26.04713531390440906 ) ) ;
#7778=EDGE_CURVE ( 'NONE', #16850, #14366, #9685, .T. ) ;
#7783=CIRCLE ( 'NONE', #7069, 0.7950200000000000600 ) ;
#7791=VERTEX_POINT ( 'NONE', #16659 ) ;
#7796=VERTEX_POINT ( 'NONE', #8131 ) ;
#7803=ADVANCED_FACE ( 'NONE', ( #4500 ), #2839, .T. ) ;
#7815=ORIENTED_EDGE ( 'NONE', *, *, #2002, .T. ) ;
#7817=VERTEX_POINT ( 'NONE', #10017 ) ;
#7828=DIRECTION ( 'NONE',  ( -0.3447671952293630548, 0.000000000000000000, -0.9386882235831439658 ) ) ;
#7831=AXIS2_PLACEMENT_3D ( 'NONE', #13840, #3768, #10730 ) ;
#7835=DIRECTION ( 'NONE',  ( -2.876946610767471886E-14, 1.000000000000000000, 2.239739066241894173E-14 ) ) ;
#7838=ORIENTED_EDGE ( 'NONE', *, *, #9225, .F. ) ;
#7841=CARTESIAN_POINT ( 'NONE',  ( 10.02683081661366593, -14.84248999999999974, -16.89519978567464165 ) ) ;
#7846=VERTEX_POINT ( 'NONE', #14697 ) ;
#7854=DIRECTION ( 'NONE',  ( -0.9964481331860212121, 0.000000000000000000, 0.08420877549337302259 ) ) ;
#7872=CARTESIAN_POINT ( 'NONE',  ( 9.907371917564091746, -3.968114999999999615, -13.23786778167655243 ) ) ;
#7894=DIRECTION ( 'NONE',  ( 0.000000000000000000, 1.000000000000000000, 0.000000000000000000 ) ) ;
#7895=LINE ( 'NONE', #16318, #11543 ) ;
#7911=ORIENTED_EDGE ( 'NONE', *, *, #18950, .F. ) ;
#7919=DIRECTION ( 'NONE',  ( 0.9636276526537417286, 0.000000000000000000, -0.2672484743474499158 ) ) ;
#7921=DIRECTION ( 'NONE',  ( 0.000000000000000000, 1.000000000000000000, 0.000000000000000000 ) ) ;
#7929=ORIENTED_EDGE ( 'NONE', *, *, #4219, .F. ) ;
#7931=EDGE_CURVE ( 'NONE', #10813, #19794, #7109, .T. ) ;
#7934=ORIENTED_EDGE ( 'NONE', *, *, #20016, .F. ) ;
#7937=VERTEX_POINT ( 'NONE', #1712 ) ;
#7954=PLANE ( 'NONE',  #17552 ) ;
#7973=CARTESIAN_POINT ( 'NONE',  ( 11.42842559562532578, 34.52875999999999834, 1.673196738795719174 ) ) ;
#7979=ORIENTED_EDGE ( 'NONE', *, *, #37, .F. ) ;
#8004=FACE_OUTER_BOUND ( 'NONE', #18550, .T. ) ;
#8006=EDGE_CURVE ( 'NONE', #7817, #8727, #14207, .T. ) ;
#8013=ORIENTED_EDGE ( 'NONE', *, *, #18142, .T. ) ;
#8023=ORIENTED_EDGE ( 'NONE', *, *, #20136, .T. ) ;
#8025=CARTESIAN_POINT ( 'NONE',  ( 19.79515554403045741, -1.983739999999999393, -10.69562145279641996 ) ) ;
#8028=CARTESIAN_POINT ( 'NONE',  ( 44.28293121686854761, -3.968114999999999615, -31.08068102505560759 ) ) ;
#8032=ORIENTED_EDGE ( 'NONE', *, *, #8006, .F. ) ;
#8049=ORIENTED_EDGE ( 'NONE', *, *, #1460, .F. ) ;
#8054=ORIENTED_EDGE ( 'NONE', *, *, #6411, .T. ) ;
#8066=FACE_OUTER_BOUND ( 'NONE', #10665, .T. ) ;
#8070=EDGE_CURVE ( 'NONE', #21386, #4038, #1558, .T. ) ;
#8072=ORIENTED_EDGE ( 'NONE', *, *, #7088, .F. ) ;
#8089=AXIS2_PLACEMENT_3D ( 'NONE', #10677, #14014, #2601 ) ;
#8097=CYLINDRICAL_SURFACE ( 'NONE', #13161, 0.7950200000000003930 ) ;
#8102=CARTESIAN_POINT ( 'NONE',  ( 10.10534066920194185, -95.96551800000000298, -14.00784516691476966 ) ) ;
#8103=VERTEX_POINT ( 'NONE', #3440 ) ;
#8113=CIRCLE ( 'NONE', #10229, 1.785937499999998179 ) ;
#8124=ADVANCED_FACE ( 'NONE', ( #15290 ), #3223, .F. ) ;
#8131=CARTESIAN_POINT ( 'NONE',  ( -47.86112874365709047, 43.41875999999999891, -23.29368419115692035 ) ) ;
#8134=DIRECTION ( 'NONE',  ( 0.000000000000000000, 1.000000000000000000, 0.000000000000000000 ) ) ;
#8142=AXIS2_PLACEMENT_3D ( 'NONE', #8572, #18956, #1937 ) ;
#8150=EDGE_CURVE ( 'NONE', #13936, #2216, #21684, .T. ) ;
#8153=AXIS2_PLACEMENT_3D ( 'NONE', #11985, #20932, #19162 ) ;
#8163=ORIENTED_EDGE ( 'NONE', *, *, #6253, .T. ) ;
#8171=EDGE_CURVE ( 'NONE', #20855, #17145, #13516, .T. ) ;
#8175=AXIS2_PLACEMENT_3D ( 'NONE', #4550, #18039, #3008 ) ;
#8180=DIRECTION ( 'NONE',  ( -0.9964481331860212121, 0.000000000000000000, 0.08420877549337302259 ) ) ;
#8181=DIRECTION ( 'NONE',  ( -0.9964481331860212121, 0.000000000000000000, 0.08420877549337300871 ) ) ;
#8201=LINE ( 'NONE', #20011, #4918 ) ;
#8203=ADVANCED_FACE ( 'NONE', ( #13731 ), #15615, .T. ) ;
#8206=CARTESIAN_POINT ( 'NONE',  ( 12.57635667311951622, 36.51313500000000545, 1.354834321244424267 ) ) ;
#8207=ORIENTED_EDGE ( 'NONE', *, *, #15365, .T. ) ;
#8211=CARTESIAN_POINT ( 'NONE',  ( 20.76310168089343478, 36.51313500000000545, -11.26763008640078212 ) ) ;
#8216=CARTESIAN_POINT ( 'NONE',  ( 9.137394532338957376, -14.84248999999999974, -13.43583653331040750 ) ) ;
#8217=DIRECTION ( 'NONE',  ( -0.9964481331860212121, 0.000000000000000000, 0.08420877549337302259 ) ) ;
#8220=DIRECTION ( 'NONE',  ( 0.6744690509234938514, -0.7360996206939018904, -0.05699866455150646993 ) ) ;
#8228=EDGE_LOOP ( 'NONE', ( #17485, #3395, #3542, #10122 ) ) ;
#8233=ORIENTED_EDGE ( 'NONE', *, *, #19106, .F. ) ;
#8245=ORIENTED_EDGE ( 'NONE', *, *, #16838, .T. ) ;
#8250=ORIENTED_EDGE ( 'NONE', *, *, #14460, .F. ) ;
#8258=ADVANCED_FACE ( 'NONE', ( #7079 ), #17252, .F. ) ;
#8260=DIRECTION ( 'NONE',  ( -0.9685006480810794960, 0.000000000000000000, -0.2490110332224836354 ) ) ;
#8267=CARTESIAN_POINT ( 'NONE',  ( -15.41509608936259035, 37.15413452960619622, -10.31276839742836415 ) ) ;
#8269=ORIENTED_EDGE ( 'NONE', *, *, #19539, .T. ) ;
#8280=ORIENTED_EDGE ( 'NONE', *, *, #9225, .T. ) ;
#8284=ORIENTED_EDGE ( 'NONE', *, *, #16836, .F. ) ;
#8288=CIRCLE ( 'NONE', #3355, 1.191259999999999319 ) ;
#8295=DIRECTION ( 'NONE',  ( 0.000000000000000000, 1.000000000000000000, 0.000000000000000000 ) ) ;
#8298=ADVANCED_FACE ( 'NONE', ( #12398 ), #15732, .F. ) ;
#8309=CARTESIAN_POINT ( 'NONE',  ( 55.52866846859686234, 34.52875999999999834, -11.12083858657437752 ) ) ;
#8315=CARTESIAN_POINT ( 'NONE',  ( -15.40791870508676631, -4.601685412415895904, -10.30897195950450573 ) ) ;
#8335=LINE ( 'NONE', #14780, #21576 ) ;
#8336=ORIENTED_EDGE ( 'NONE', *, *, #8842, .T. ) ;
#8340=ORIENTED_EDGE ( 'NONE', *, *, #16884, .F. ) ;
#8348=VECTOR ( 'NONE', #10940, 1000.000000000000114 ) ;
#8353=ORIENTED_EDGE ( 'NONE', *, *, #10185, .F. ) ;
#8354=ORIENTED_EDGE ( 'NONE', *, *, #16026, .T. ) ;
#8355=DIRECTION ( 'NONE',  ( -0.2490110332224836354, 0.000000000000000000, 0.9685006480810794960 ) ) ;
#8361=LINE ( 'NONE', #3176, #2233 ) ;
#8369=CYLINDRICAL_SURFACE ( 'NONE', #1861, 0.7950200000000003930 ) ;
#8389=DIRECTION ( 'NONE',  ( 0.08420877549337300871, 0.000000000000000000, 0.9964481331860212121 ) ) ;
#8393=PLANE ( 'NONE',  #11013 ) ;
#8396=ORIENTED_EDGE ( 'NONE', *, *, #10058, .F. ) ;
#8399=VERTEX_POINT ( 'NONE', #9280 ) ;
#8412=EDGE_CURVE ( 'NONE', #18743, #11237, #16055, .T. ) ;
#8423=DIRECTION ( 'NONE',  ( -0.000000000000000000, -1.000000000000000000, 0.000000000000000000 ) ) ;
#8425=CARTESIAN_POINT ( 'NONE',  ( 12.02474915109715603, -1.983739999999999393, -13.51434638588835391 ) ) ;
#8437=CIRCLE ( 'NONE', #3916, 0.7950200000000000600 ) ;
#8448=ORIENTED_EDGE ( 'NONE', *, *, #5349, .F. ) ;
#8454=CARTESIAN_POINT ( 'NONE',  ( -18.18961309330695997, -3.266559801243759331, -25.80119252674831998 ) ) ;
#8462=VERTEX_POINT ( 'NONE', #16158 ) ;
#8470=CARTESIAN_POINT ( 'NONE',  ( 14.05820270259704152, 36.51313500000000545, -15.03781736451272444 ) ) ;
#8477=SURFACE_SIDE_STYLE ('',( #2060 ) ) ;
#8478=CARTESIAN_POINT ( 'NONE',  ( 9.335363283976800375, 34.52875999999999834, -14.20581391854862474 ) ) ;
#8490=ORIENTED_EDGE ( 'NONE', *, *, #11017, .T. ) ;
#8495=AXIS2_PLACEMENT_3D ( 'NONE', #21187, #9364, #12695 ) ;
#8496=DIRECTION ( 'NONE',  ( -0.000000000000000000, -1.000000000000000000, 0.000000000000000000 ) ) ;
#8503=DIRECTION ( 'NONE',  ( -0.000000000000000000, -1.000000000000000000, 0.000000000000000000 ) ) ;
#8506=AXIS2_PLACEMENT_3D ( 'NONE', #3906, #7431, #5781 ) ;
#8507=CARTESIAN_POINT ( 'NONE',  ( 21.25660046192028929, 34.52875999999999834, -13.18703856829094079 ) ) ;
#8522=LINE ( 'NONE', #3673, #11280 ) ;
#8527=VECTOR ( 'NONE', #15265, 1000.000000000000000 ) ;
#8530=FACE_OUTER_BOUND ( 'NONE', #14003, .T. ) ;
#8538=CARTESIAN_POINT ( 'NONE',  ( 17.02725982432203367, 128.5105379999999968, -14.27444360421403857 ) ) ;
#8546=DIRECTION ( 'NONE',  ( -0.08420877549337300871, 0.000000000000000000, -0.9964481331860212121 ) ) ;
#8548=DIRECTION ( 'NONE',  ( 0.000000000000000000, 1.000000000000000000, 0.000000000000000000 ) ) ;
#8551=EDGE_CURVE ( 'NONE', #6728, #3226, #1826, .T. ) ;
#8565=EDGE_CURVE ( 'NONE', #21482, #21386, #2188, .T. ) ;
#8566=VERTEX_POINT ( 'NONE', #8703 ) ;
#8570=AXIS2_PLACEMENT_3D ( 'NONE', #18808, #6881, #11754 ) ;
#8572=CARTESIAN_POINT ( 'NONE',  ( 12.02474915109715603, -3.968114999999999615, -13.51434638588835391 ) ) ;
#8576=ORIENTED_EDGE ( 'NONE', *, *, #17803, .T. ) ;
#8591=CARTESIAN_POINT ( 'NONE',  ( 55.81697695389291169, 36.51313500000000545, -11.14520323105768362 ) ) ;
#8592=FILL_AREA_STYLE_COLOUR ( '', #13514 ) ;
#8596=VECTOR ( 'NONE', #5400, 1000.000000000000000 ) ;
#8606=ORIENTED_EDGE ( 'NONE', *, *, #16985, .T. ) ;
#8609=DIRECTION ( 'NONE',  ( -0.7334850928793773539, 0.6768732144311022658, 0.06198604769976947398 ) ) ;
#8612=CARTESIAN_POINT ( 'NONE',  ( 36.54633153140314761, 36.51313500000000545, -9.516661413425623550 ) ) ;
#8615=CARTESIAN_POINT ( 'NONE',  ( 17.02725982432203367, 128.5105379999999968, -14.27444360421403857 ) ) ;
#8623=ORIENTED_EDGE ( 'NONE', *, *, #6927, .T. ) ;
#8628=ORIENTED_EDGE ( 'NONE', *, *, #13864, .T. ) ;
#8629=VECTOR ( 'NONE', #5843, 1000.000000000000000 ) ;
#8630=ORIENTED_EDGE ( 'NONE', *, *, #4141, .T. ) ;
#8649=EDGE_CURVE ( 'NONE', #4259, #6430, #8929, .T. ) ;
#8656=ORIENTED_EDGE ( 'NONE', *, *, #9518, .F. ) ;
#8658=VECTOR ( 'NONE', #3622, 1000.000000000000000 ) ;
#8668=DIRECTION ( 'NONE',  ( 0.2490110332224846623, 0.000000000000000000, -0.9685006480810793850 ) ) ;
#8671=EDGE_CURVE ( 'NONE', #9683, #9903, #5172, .T. ) ;
#8682=PLANE ( 'NONE',  #18991 ) ;
#8686=EDGE_CURVE ( 'NONE', #13702, #6259, #201, .T. ) ;
#8689=CARTESIAN_POINT ( 'NONE',  ( 44.28293121686854761, 36.51313500000000545, -31.08068102505560759 ) ) ;
#8692=ORIENTED_EDGE ( 'NONE', *, *, #14371, .F. ) ;
#8694=DIRECTION ( 'NONE',  ( 0.000000000000000000, 1.000000000000000000, 0.000000000000000000 ) ) ;
#8700=VERTEX_POINT ( 'NONE', #10378 ) ;
#8703=CARTESIAN_POINT ( 'NONE',  ( 12.79472653632228507, 34.52875999999999834, -13.31637763425449883 ) ) ;
#8709=AXIS2_PLACEMENT_3D ( 'NONE', #19336, #17914, #2760 ) ;
#8714=ADVANCED_FACE ( 'NONE', ( #8808 ), #18982, .T. ) ;
#8716=EDGE_CURVE ( 'NONE', #18111, #13681, #12410, .T. ) ;
#8727=VERTEX_POINT ( 'NONE', #20859 ) ;
#8738=CARTESIAN_POINT ( 'NONE',  ( -19.26432987443570966, -5.953760000000000829, -73.22178168742661342 ) ) ;
#8753=DIRECTION ( 'NONE',  ( -0.9685006480810794960, 0.000000000000000000, -0.2490110332224836354 ) ) ;
#8758=DIRECTION ( 'NONE',  ( -0.000000000000000000, -1.000000000000000000, 0.000000000000000000 ) ) ;
#8776=ORIENTED_EDGE ( 'NONE', *, *, #362, .F. ) ;
#8783=ORIENTED_EDGE ( 'NONE', *, *, #8150, .T. ) ;
#8788=EDGE_CURVE ( 'NONE', #9986, #14245, #17562, .T. ) ;
#8794=LINE ( 'NONE', #12354, #15766 ) ;
#8798=CIRCLE ( 'NONE', #16249, 0.7950200000000000600 ) ;
#8799=CARTESIAN_POINT ( 'NONE',  ( 17.30373842852263877, 34.52875999999999834, -12.15706637069277107 ) ) ;
#8808=FACE_OUTER_BOUND ( 'NONE', #12667, .T. ) ;
#8812=EDGE_CURVE ( 'NONE', #12648, #7062, #13467, .T. ) ;
#8815=VERTEX_POINT ( 'NONE', #19207 ) ;
#8817=EDGE_CURVE ( 'NONE', #3064, #1375, #12762, .T. ) ;
#8822=CIRCLE ( 'NONE', #3500, 0.7950200000000000600 ) ;
#8823=LINE ( 'NONE', #438, #15969 ) ;
#8833=CARTESIAN_POINT ( 'NONE',  ( 62.90077106633562209, -14.84248999999999974, 8.141649473166729933 ) ) ;
#8835=CYLINDRICAL_SURFACE ( 'NONE', #317, 11.02160133116777452 ) ;
#8836=ORIENTED_EDGE ( 'NONE', *, *, #16985, .F. ) ;
#8841=VERTEX_POINT ( 'NONE', #19542 ) ;
#8842=EDGE_CURVE ( 'NONE', #15164, #21307, #12928, .T. ) ;
#8848=VECTOR ( 'NONE', #7727, 1000.000000000000114 ) ;
#8859=DIRECTION ( 'NONE',  ( -0.08420877549337302259, 0.000000000000000000, -0.9964481331860212121 ) ) ;
#8862=AXIS2_PLACEMENT_3D ( 'NONE', #10262, #5176, #17129 ) ;
#8866=EDGE_CURVE ( 'NONE', #12465, #171, #4177, .T. ) ;
#8872=EDGE_LOOP ( 'NONE', ( #10395, #3194, #6579, #4610 ) ) ;
#8874=LINE ( 'NONE', #12313, #16979 ) ;
#8875=( BOUNDED_CURVE ( )  B_SPLINE_CURVE ( 3, ( #16734, #8315, #21798, #6652 ),
 .UNSPECIFIED., .F., .F. ) 
 B_SPLINE_CURVE_WITH_KNOTS ( ( 4, 4 ),
 ( 2.992738460178339999, 3.006667970820978031 ),
 .UNSPECIFIED. ) 
 CURVE ( )  GEOMETRIC_REPRESENTATION_ITEM ( )  RATIONAL_B_SPLINE_CURVE ( ( 1.000000000000000000, 0.9999838307931325776, 0.9999838307931325776, 1.000000000000000000 ) ) 
 REPRESENTATION_ITEM ( '' )  );
#8885=CARTESIAN_POINT ( 'NONE',  ( 17.30373842852263877, -1.983739999999999393, -12.15706637069277107 ) ) ;
#8893=CARTESIAN_POINT ( 'NONE',  ( -51.84716326864270286, 38.25938500000000175, -70.46824097531958842 ) ) ;
#8899=FACE_OUTER_BOUND ( 'NONE', #6239, .T. ) ;
#8906=ORIENTED_EDGE ( 'NONE', *, *, #3020, .T. ) ;
#8917=CIRCLE ( 'NONE', #8570, 3.970019999999999438 ) ;
#8919=DIRECTION ( 'NONE',  ( 0.000000000000000000, 1.000000000000000000, 0.000000000000000000 ) ) ;
#8921=DIRECTION ( 'NONE',  ( 0.000000000000000000, 1.000000000000000000, 0.000000000000000000 ) ) ;
#8924=ORIENTED_EDGE ( 'NONE', *, *, #21796, .T. ) ;
#8929=LINE ( 'NONE', #5497, #12084 ) ;
#8933=VECTOR ( 'NONE', #4425, 1000.000000000000114 ) ;
#8939=DIRECTION ( 'NONE',  ( 0.000000000000000000, -1.000000000000000000, 0.000000000000000000 ) ) ;
#8949=VERTEX_POINT ( 'NONE', #18312 ) ;
#8950=VERTEX_POINT ( 'NONE', #4932 ) ;
#8953=AXIS2_PLACEMENT_3D ( 'NONE', #3617, #11802, #5479 ) ;
#8958=ORIENTED_EDGE ( 'NONE', *, *, #6753, .F. ) ;
#8965=PLANE ( 'NONE',  #1540 ) ;
#8967=CIRCLE ( 'NONE', #21327, 3.970020000000000326 ) ;
#8975=CARTESIAN_POINT ( 'NONE',  ( 46.03750000000000142, -14.84248999999999974, -10.31874999999999964 ) ) ;
#8990=DIRECTION ( 'NONE',  ( 0.2490110332224846623, 0.000000000000000000, -0.9685006480810793850 ) ) ;
#8992=ORIENTED_EDGE ( 'NONE', *, *, #1932, .T. ) ;
#9003=EDGE_LOOP ( 'NONE', ( #4783, #11145, #10484, #7815 ) ) ;
#9019=ORIENTED_EDGE ( 'NONE', *, *, #8788, .F. ) ;
#9026=DIRECTION ( 'NONE',  ( 0.08420877549337300871, 0.000000000000000000, 0.9964481331860212121 ) ) ;
#9030=FACE_OUTER_BOUND ( 'NONE', #18319, .T. ) ;
#9040=ORIENTED_EDGE ( 'NONE', *, *, #15467, .T. ) ;
#9046=CARTESIAN_POINT ( 'NONE',  ( 12.02474915109715603, -95.96551800000000298, -13.51434638588835391 ) ) ;
#9054=ORIENTED_EDGE ( 'NONE', *, *, #6753, .T. ) ;
#9084=PLANE ( 'NONE',  #18059 ) ;
#9114=ORIENTED_EDGE ( 'NONE', *, *, #19973, .T. ) ;
#9128=PRODUCT_DEFINITION_FORMATION_WITH_SPECIFIED_SOURCE ( 'ANY', '', #4914, .NOT_KNOWN. ) ;
#9129=DIRECTION ( 'NONE',  ( -0.6744690509234934073, -0.7360996206939023345, 0.05699866455150641442 ) ) ;
#9130=DIRECTION ( 'NONE',  ( 0.000000000000000000, 1.000000000000000000, 0.000000000000000000 ) ) ;
#9135=EDGE_LOOP ( 'NONE', ( #6741, #19562, #3990, #17088 ) ) ;
#9146=ORIENTED_EDGE ( 'NONE', *, *, #14923, .T. ) ;
#9149=PLANE ( 'NONE',  #12437 ) ;
#9150=AXIS2_PLACEMENT_3D ( 'NONE', #7317, #5651, #4109 ) ;
#9152=DIRECTION ( 'NONE',  ( -0.2490110332224836354, 0.000000000000000000, 0.9685006480810794960 ) ) ;
#9166=ORIENTED_EDGE ( 'NONE', *, *, #16484, .T. ) ;
#9172=AXIS2_PLACEMENT_3D ( 'NONE', #18282, #13115, #18188 ) ;
#9186=DIRECTION ( 'NONE',  ( 0.7334850928793772429, 0.6768732144311025989, -0.06198604769976985562 ) ) ;
#9187=CARTESIAN_POINT ( 'NONE',  ( -24.21104940531825633, -10.87373999999999974, -25.29232732678598339 ) ) ;
#9190=CARTESIAN_POINT ( 'NONE',  ( -46.55710204590916135, -5.714364999999999029, -7.870588902259476605 ) ) ;
#9192=ORIENTED_EDGE ( 'NONE', *, *, #5473, .T. ) ;
#9219=DIRECTION ( 'NONE',  ( -0.9964481331860213231, 0.000000000000000000, 0.08420877549337311974 ) ) ;
#9223=DIRECTION ( 'NONE',  ( 0.08420877549337300871, 0.000000000000000000, 0.9964481331860212121 ) ) ;
#9225=EDGE_CURVE ( 'NONE', #11084, #171, #5311, .T. ) ;
#9228=LINE ( 'NONE', #12791, #3573 ) ;
#9229=ORIENTED_EDGE ( 'NONE', *, *, #9813, .F. ) ;
#9233=VECTOR ( 'NONE', #14619, 1000.000000000000000 ) ;
#9241=DIRECTION ( 'NONE',  ( -0.9964481331860213231, 0.000000000000000000, 0.08420877549337306422 ) ) ;
#9244=CARTESIAN_POINT ( 'NONE',  ( 11.75439013559175017, 128.5105379999999968, 4.331204221326972359 ) ) ;
#9245=DIRECTION ( 'NONE',  ( 0.000000000000000000, 1.000000000000000000, 0.000000000000000000 ) ) ;
#9250=EDGE_CURVE ( 'NONE', #13702, #1, #17092, .T. ) ;
#9256=ORIENTED_EDGE ( 'NONE', *, *, #13734, .F. ) ;
#9270=ORIENTED_EDGE ( 'NONE', *, *, #639, .F. ) ;
#9273=DIRECTION ( 'NONE',  ( -0.9685006480810792739, 0.000000000000000000, -0.2490110332224846346 ) ) ;
#9280=CARTESIAN_POINT ( 'NONE',  ( 56.47666780297049627, 34.52875999999999834, 1.109116340531466127 ) ) ;
#9313=PLANE ( 'NONE',  #18662 ) ;
#9314=ORIENTED_EDGE ( 'NONE', *, *, #11413, .T. ) ;
#9324=CIRCLE ( 'NONE', #18855, 0.7950200000000000600 ) ;
#9327=ADVANCED_FACE ( 'NONE', ( #14129 ), #17868, .T. ) ;
#9331=CARTESIAN_POINT ( 'NONE',  ( -46.55773479047372376, -10.87373999999999974, -7.870535429687039120 ) ) ;
#9343=DIRECTION ( 'NONE',  ( -0.2672484743474505819, 0.000000000000000000, -0.9636276526537416176 ) ) ;
#9344=ORIENTED_EDGE ( 'NONE', *, *, #20842, .T. ) ;
#9345=CARTESIAN_POINT ( 'NONE',  ( -19.99570496368815142, -9.590920198756240467, -10.11526441440630286 ) ) ;
#9353=EDGE_CURVE ( 'NONE', #6731, #13482, #9228, .T. ) ;
#9355=LINE ( 'NONE', #16122, #15460 ) ;
#9356=ORIENTED_EDGE ( 'NONE', *, *, #16700, .F. ) ;
#9359=DIRECTION ( 'NONE',  ( -0.4857267349359799535, 0.000000000000000000, 0.8741107132214044340 ) ) ;
#9362=CARTESIAN_POINT ( 'NONE',  ( -14.99341658050716930, 36.73131074634049753, -10.07873794320098426 ) ) ;
#9364=DIRECTION ( 'NONE',  ( 0.000000000000000000, 1.000000000000000000, 0.000000000000000000 ) ) ;
#9368=ORIENTED_EDGE ( 'NONE', *, *, #15943, .T. ) ;
#9369=EDGE_CURVE ( 'NONE', #18111, #1622, #722, .T. ) ;
#9371=VERTEX_POINT ( 'NONE', #19514 ) ;
#9374=FACE_OUTER_BOUND ( 'NONE', #3281, .T. ) ;
#9375=LINE ( 'NONE', #17798, #5798 ) ;
#9380=CARTESIAN_POINT ( 'NONE',  ( 11.11006317807338561, -14.84248999999999974, 0.5252656612939419212 ) ) ;
#9397=EDGE_CURVE ( 'NONE', #4458, #6182, #11116, .T. ) ;
#9409=CIRCLE ( 'NONE', #16827, 5.158739999999999881 ) ;
#9421=DIRECTION ( 'NONE',  ( -0.7334850928793772429, -0.6768732144311025989, 0.06198604769976985562 ) ) ;
#9423=ORIENTED_EDGE ( 'NONE', *, *, #8006, .T. ) ;
#9427=DIRECTION ( 'NONE',  ( 0.000000000000000000, 1.000000000000000000, 0.000000000000000000 ) ) ;
#9434=LINE ( 'NONE', #18866, #11843 ) ;
#9443=CARTESIAN_POINT ( 'NONE',  ( 3.360635606688116894, -3.968114999999999615, -20.45316710734507026 ) ) ;
#9447=DIRECTION ( 'NONE',  ( -0.000000000000000000, -1.000000000000000000, 0.000000000000000000 ) ) ;
#9448=ORIENTED_EDGE ( 'NONE', *, *, #1563, .F. ) ;
#9452=ORIENTED_EDGE ( 'NONE', *, *, #17264, .T. ) ;
#9455=VECTOR ( 'NONE', #20653, 1000.000000000000114 ) ;
#9465=DIRECTION ( 'NONE',  ( 0.000000000000000000, 1.000000000000000000, 0.000000000000000000 ) ) ;
#9466=VERTEX_POINT ( 'NONE', #11003 ) ;
#9467=ORIENTED_EDGE ( 'NONE', *, *, #2472, .F. ) ;
#9472=EDGE_LOOP ( 'NONE', ( #7251, #8032, #13260, #9763 ) ) ;
#9480=DIRECTION ( 'NONE',  ( 0.08420877549337300871, 0.000000000000000000, 0.9964481331860212121 ) ) ;
#9482=DIRECTION ( 'NONE',  ( -0.5285133232210438292, 0.8477492467026710443, 0.04466410071749180727 ) ) ;
#9485=ORIENTED_EDGE ( 'NONE', *, *, #8686, .F. ) ;
#9486=LINE ( 'NONE', #21096, #9642 ) ;
#9502=VECTOR ( 'NONE', #12148, 1000.000000000000000 ) ;
#9504=ADVANCED_FACE ( 'NONE', ( #16751 ), #18388, .F. ) ;
#9506=AXIS2_PLACEMENT_3D ( 'NONE', #7258, #19180, #20609 ) ;
#9518=EDGE_CURVE ( 'NONE', #17468, #12588, #8335, .T. ) ;
#9531=ORIENTED_EDGE ( 'NONE', *, *, #2720, .T. ) ;
#9534=CARTESIAN_POINT ( 'NONE',  ( 18.07371581377308800, -1.983739999999999393, -11.95909761906105473 ) ) ;
#9549=DIRECTION ( 'NONE',  ( -0.9685006480810794960, 0.000000000000000000, -0.2490110332224836354 ) ) ;
#9552=CARTESIAN_POINT ( 'NONE',  ( 28.56548256563643662, 36.51313500000000545, -12.12873025803960658 ) ) ;
#9555=AXIS2_PLACEMENT_3D ( 'NONE', #21160, #21381, #7579 ) ;
#9562=VECTOR ( 'NONE', #10000, 1000.000000000000114 ) ;
#9564=VERTEX_POINT ( 'NONE', #3146 ) ;
#9573=ORIENTED_EDGE ( 'NONE', *, *, #20748, .T. ) ;
#9581=VERTEX_POINT ( 'NONE', #18285 ) ;
#9583=ORIENTED_EDGE ( 'NONE', *, *, #3508, .F. ) ;
#9585=EDGE_LOOP ( 'NONE', ( #10385, #17245, #16552, #10834 ) ) ;
#9599=CARTESIAN_POINT ( 'NONE',  ( -15.39353573898878658, -2.254660308866960339, -10.30107656633069979 ) ) ;
#9601=CARTESIAN_POINT ( 'NONE',  ( -49.72082486877479113, 38.25938500000000175, -7.603226040068017610 ) ) ;
#9602=FACE_OUTER_BOUND ( 'NONE', #21424, .T. ) ;
#9604=ORIENTED_EDGE ( 'NONE', *, *, #8649, .F. ) ;
#9615=CIRCLE ( 'NONE', #17768, 1.785937499999998179 ) ;
#9642=VECTOR ( 'NONE', #19654, 1000.000000000000114 ) ;
#9644=DIRECTION ( 'NONE',  ( -0.9685006480810792739, 0.000000000000000000, -0.2490110332224846346 ) ) ;
#9657=CIRCLE ( 'NONE', #16727, 11.02160133116777985 ) ;
#9658=CARTESIAN_POINT ( 'NONE',  ( 65.04486224192415023, -1.983739999999999393, -32.83524980818705785 ) ) ;
#9661=CARTESIAN_POINT ( 'NONE',  ( -15.41509608936259035, 37.15413452960619622, -10.31276839742836415 ) ) ;
#9672=VECTOR ( 'NONE', #4542, 1000.000000000000000 ) ;
#9683=VERTEX_POINT ( 'NONE', #10319 ) ;
#9685=LINE ( 'NONE', #12922, #6392 ) ;
#9701=FACE_OUTER_BOUND ( 'NONE', #113, .T. ) ;
#9704=CARTESIAN_POINT ( 'NONE',  ( -46.55773479047372376, 38.26001999999999725, -7.870535429687039120 ) ) ;
#9708=CARTESIAN_POINT ( 'NONE',  ( 19.99312429566830218, 34.52875999999999834, -11.46559883803463720 ) ) ;
#9714=VERTEX_POINT ( 'NONE', #366 ) ;
#9725=DIRECTION ( 'NONE',  ( -0.08420877549337300871, 0.000000000000000000, -0.9964481331860212121 ) ) ;
#9747=ADVANCED_FACE ( 'NONE', ( #16849 ), #255, .T. ) ;
#9758=DIRECTION ( 'NONE',  ( 0.9685006480810794960, 0.000000000000000000, 0.2490110332224836354 ) ) ;
#9762=CYLINDRICAL_SURFACE ( 'NONE', #21413, 0.7950200000000000600 ) ;
#9763=ORIENTED_EDGE ( 'NONE', *, *, #15205, .T. ) ;
#9782=AXIS2_PLACEMENT_3D ( 'NONE', #12582, #9130, #9241 ) ;
#9783=VERTEX_POINT ( 'NONE', #13545 ) ;
#9798=CIRCLE ( 'NONE', #16192, 3.970019999999997662 ) ;
#9804=CARTESIAN_POINT ( 'NONE',  ( 12.57635667311951622, -95.96551800000000298, 1.354834321244424267 ) ) ;
#9808=AXIS2_PLACEMENT_3D ( 'NONE', #14189, #7637, #20897 ) ;
#9813=EDGE_CURVE ( 'NONE', #16186, #10813, #19351, .T. ) ;
#9814=DIRECTION ( 'NONE',  ( -0.000000000000000000, -1.000000000000000000, 0.000000000000000000 ) ) ;
#9819=DIRECTION ( 'NONE',  ( 0.000000000000000000, 1.000000000000000000, 0.000000000000000000 ) ) ;
#9824=AXIS2_PLACEMENT_3D ( 'NONE', #20221, #21882, #19903 ) ;
#9830=VERTEX_POINT ( 'NONE', #4971 ) ;
#9832=LINE ( 'NONE', #13726, #5709 ) ;
#9861=ORIENTED_EDGE ( 'NONE', *, *, #20170, .T. ) ;
#9863=CYLINDRICAL_SURFACE ( 'NONE', #19999, 1.785937499999999512 ) ;
#9867=CARTESIAN_POINT ( 'NONE',  ( -47.86049599909252805, 38.25938500000000175, -23.29373766372935961 ) ) ;
#9873=LINE ( 'NONE', #21388, #14804 ) ;
#9874=ORIENTED_EDGE ( 'NONE', *, *, #7461, .T. ) ;
#9879=EDGE_LOOP ( 'NONE', ( #13562, #8396, #9270, #15330 ) ) ;
#9888=VERTEX_POINT ( 'NONE', #4869 ) ;
#9891=CIRCLE ( 'NONE', #1029, 3.970019999999997662 ) ;
#9902=VECTOR ( 'NONE', #4284, 1000.000000000000000 ) ;
#9903=VERTEX_POINT ( 'NONE', #16389 ) ;
#9909=ORIENTED_EDGE ( 'NONE', *, *, #339, .F. ) ;
#9920=ORIENTED_EDGE ( 'NONE', *, *, #17505, .F. ) ;
#9922=AXIS2_PLACEMENT_3D ( 'NONE', #17538, #9447, #19293 ) ;
#9926=LINE ( 'NONE', #3312, #19379 ) ;
#9928=ORIENTED_EDGE ( 'NONE', *, *, #11297, .F. ) ;
#9932=CARTESIAN_POINT ( 'NONE',  ( 46.03750000000000142, 34.52875999999999834, -10.31874999999999964 ) ) ;
#9940=AXIS2_PLACEMENT_3D ( 'NONE', #8833, #3654, #18896 ) ;
#9942=ADVANCED_FACE ( 'NONE', ( #11502 ), #6535, .T. ) ;
#9956=PLANE ( 'NONE',  #9824 ) ;
#9957=VECTOR ( 'NONE', #14275, 1000.000000000000000 ) ;
#9967=CARTESIAN_POINT ( 'NONE',  ( -21.29909891687151813, -9.590920198756240467, -25.53841317587618320 ) ) ;
#9986=VERTEX_POINT ( 'NONE', #12272 ) ;
#9989=CARTESIAN_POINT ( 'NONE',  ( -16.07247711516169275, -5.309201820043501385, -10.44681224123558039 ) ) ;
#10000=DIRECTION ( 'NONE',  ( 0.9685006480810792739, 0.000000000000000000, 0.2490110332224846346 ) ) ;
#10001=VERTEX_POINT ( 'NONE', #13504 ) ;
#10002=VECTOR ( 'NONE', #10188, 1000.000000000000000 ) ;
#10013=CIRCLE ( 'NONE', #488, 0.7950200000000003930 ) ;
#10017=CARTESIAN_POINT ( 'NONE',  ( 59.61686353177688602, 34.52875999999999834, -0.7993558564620834028 ) ) ;
#10029=ADVANCED_FACE ( 'NONE', ( #13723 ), #3429, .T. ) ;
#10037=VECTOR ( 'NONE', #269, 1000.000000000000114 ) ;
#10043=PRESENTATION_STYLE_ASSIGNMENT (( #1852 ) ) ;
#10044=PLANE ( 'NONE',  #19025 ) ;
#10052=ORIENTED_EDGE ( 'NONE', *, *, #5945, .F. ) ;
#10058=EDGE_CURVE ( 'NONE', #5959, #16695, #6856, .T. ) ;
#10064=CARTESIAN_POINT ( 'NONE',  ( 3.805353748838121053, -3.968114999999999615, -22.18284873352824960 ) ) ;
#10070=CARTESIAN_POINT ( 'NONE',  ( 17.22522857595987844, -3.968114999999999615, -15.04442098945225403 ) ) ;
#10072=EDGE_LOOP ( 'NONE', ( #5790, #16319, #7054, #16363 ) ) ;
#10095=CYLINDRICAL_SURFACE ( 'NONE', #21070, 0.7950200000000003930 ) ;
#10102=DIRECTION ( 'NONE',  ( -0.2490110332224846623, 0.000000000000000000, 0.9685006480810793850 ) ) ;
#10104=CARTESIAN_POINT ( 'NONE',  ( -14.45909654372122688, -3.968114999999678538, -9.781826438796198175 ) ) ;
#10116=DIRECTION ( 'NONE',  ( 0.000000000000000000, 1.000000000000000000, 0.000000000000000000 ) ) ;
#10122=ORIENTED_EDGE ( 'NONE', *, *, #10218, .F. ) ;
#10124=EDGE_CURVE ( 'NONE', #4031, #10557, #5514, .T. ) ;
#10125=DIRECTION ( 'NONE',  ( -0.9964481331860212121, 0.000000000000000000, 0.08420877549337302259 ) ) ;
#10139=ORIENTED_EDGE ( 'NONE', *, *, #16412, .F. ) ;
#10140=DIRECTION ( 'NONE',  ( -0.2490110332224857170, 0.000000000000000000, 0.9685006480810790519 ) ) ;
#10155=ORIENTED_EDGE ( 'NONE', *, *, #18480, .F. ) ;
#10157=DIRECTION ( 'NONE',  ( -0.08420877549337300871, 0.000000000000000000, -0.9964481331860212121 ) ) ;
#10165=( BOUNDED_CURVE ( )  B_SPLINE_CURVE ( 3, ( #17785, #2633, #9362, #16129 ),
 .UNSPECIFIED., .F., .T. ) 
 B_SPLINE_CURVE_WITH_KNOTS ( ( 4, 4 ),
 ( 4.712388980384104364, 5.524536188664038505 ),
 .UNSPECIFIED. ) 
 CURVE ( )  GEOMETRIC_REPRESENTATION_ITEM ( )  RATIONAL_B_SPLINE_CURVE ( ( 1.000000000000000000, 0.9457858982560934935, 0.9457858982560934935, 1.000000000000000000 ) ) 
 REPRESENTATION_ITEM ( '' )  );
#10166=VERTEX_POINT ( 'NONE', #18976 ) ;
#10168=DIRECTION ( 'NONE',  ( -0.9685006480810793850, 0.000000000000000000, -0.2490110332224846623 ) ) ;
#10171=VERTEX_POINT ( 'NONE', #15805 ) ;
#10175=ADVANCED_FACE ( 'NONE', ( #9030 ), #1066, .T. ) ;
#10177=AXIS2_PLACEMENT_3D ( 'NONE', #11508, #4978, #3110 ) ;
#10185=EDGE_CURVE ( 'NONE', #5344, #1525, #9798, .T. ) ;
#10188=DIRECTION ( 'NONE',  ( 0.000000000000000000, 1.000000000000000000, 0.000000000000000000 ) ) ;
#10192=CARTESIAN_POINT ( 'NONE',  ( -19.26432987443570966, 38.49878000000000355, -73.22178168742661342 ) ) ;
#10206=VERTEX_POINT ( 'NONE', #2629 ) ;
#10208=CARTESIAN_POINT ( 'NONE',  ( 3.805353748838121053, -3.968114999999999615, -22.18284873352824960 ) ) ;
#10210=CIRCLE ( 'NONE', #680, 0.7950200000000000600 ) ;
#10212=CIRCLE ( 'NONE', #9506, 1.983739999999995396 ) ;
#10213=ORIENTED_EDGE ( 'NONE', *, *, #15360, .T. ) ;
#10218=EDGE_CURVE ( 'NONE', #19233, #14947, #6267, .T. ) ;
#10229=AXIS2_PLACEMENT_3D ( 'NONE', #3001, #21022, #14405 ) ;
#10236=VECTOR ( 'NONE', #12403, 1000.000000000000000 ) ;
#10252=CARTESIAN_POINT ( 'NONE',  ( 3.360635606688116894, -1.983739999999999393, -20.45316710734507026 ) ) ;
#10262=CARTESIAN_POINT ( 'NONE',  ( 46.03750000000000142, -14.84248999999999974, -10.31874999999999964 ) ) ;
#10288=VECTOR ( 'NONE', #4982, 1000.000000000000114 ) ;
#10299=( BOUNDED_CURVE ( )  B_SPLINE_CURVE ( 3, ( #15106, #3148, #10104, #258 ),
 .UNSPECIFIED., .F., .F. ) 
 B_SPLINE_CURVE_WITH_KNOTS ( ( 4, 4 ),
 ( 0.7586491185162420603, 1.570796326795481868 ),
 .UNSPECIFIED. ) 
 CURVE ( )  GEOMETRIC_REPRESENTATION_ITEM ( )  RATIONAL_B_SPLINE_CURVE ( ( 1.000000000000000000, 0.9457858982561848649, 0.9457858982561848649, 1.000000000000000000 ) ) 
 REPRESENTATION_ITEM ( '' )  );
#10317=CARTESIAN_POINT ( 'NONE',  ( 9.335363283976800375, -3.968114999999999615, -14.20581391854862474 ) ) ;
#10319=CARTESIAN_POINT ( 'NONE',  ( 9.907371917564091746, 34.52875999999999834, -13.23786778167655243 ) ) ;
#10321=EDGE_CURVE ( 'NONE', #12395, #6616, #14465, .T. ) ;
#10322=CARTESIAN_POINT ( 'NONE',  ( 17.22522857595987844, 34.52875999999999834, -15.04442098945225403 ) ) ;
#10331=ADVANCED_FACE ( 'NONE', ( #15917 ), #12586, .T. ) ;
#10336=DIRECTION ( 'NONE',  ( 0.9685006480810793850, 0.000000000000000000, 0.2490110332224846623 ) ) ;
#10345=CYLINDRICAL_SURFACE ( 'NONE', #17765, 0.7950200000000000600 ) ;
#10346=VECTOR ( 'NONE', #11314, 1000.000000000000000 ) ;
#10349=ORIENTED_EDGE ( 'NONE', *, *, #15086, .T. ) ;
#10351=EDGE_CURVE ( 'NONE', #6373, #9830, #10915, .T. ) ;
#10358=LINE ( 'NONE', #16878, #5412 ) ;
#10367=ORIENTED_EDGE ( 'NONE', *, *, #7778, .F. ) ;
#10369=LINE ( 'NONE', #414, #18089 ) ;
#10373=AXIS2_PLACEMENT_3D ( 'NONE', #902, #13184, #1324 ) ;
#10378=CARTESIAN_POINT ( 'NONE',  ( 12.25799425556778388, -3.968114999999999615, 0.2069032437451798767 ) ) ;
#10382=EDGE_LOOP ( 'NONE', ( #20615, #9485, #3746, #20326 ) ) ;
#10385=ORIENTED_EDGE ( 'NONE', *, *, #16956, .T. ) ;
#10392=CARTESIAN_POINT ( 'NONE',  ( 9.256853431388732290, 36.51313500000000545, -17.09316853730597074 ) ) ;
#10395=ORIENTED_EDGE ( 'NONE', *, *, #10321, .F. ) ;
#10397=VECTOR ( 'NONE', #9644, 1000.000000000000114 ) ;
#10398=DIRECTION ( 'NONE',  ( -0.2672484743474491942, 0.000000000000000000, -0.9636276526537419507 ) ) ;
#10408=ORIENTED_EDGE ( 'NONE', *, *, #12589, .T. ) ;
#10450=CARTESIAN_POINT ( 'NONE',  ( -53.00154558624916490, -5.714999999999999858, -22.85927301266823264 ) ) ;
#10462=CARTESIAN_POINT ( 'NONE',  ( -28.19602381335591801, -6.905625000000000568, -72.46697370030818774 ) ) ;
#10464=DIRECTION ( 'NONE',  ( -0.2490110332224857170, 0.000000000000000000, 0.9685006480810790519 ) ) ;
#10465=VERTEX_POINT ( 'NONE', #11954 ) ;
#10479=VERTEX_POINT ( 'NONE', #20230 ) ;
#10484=ORIENTED_EDGE ( 'NONE', *, *, #4141, .F. ) ;
#10489=ORIENTED_EDGE ( 'NONE', *, *, #18409, .F. ) ;
#10494=CARTESIAN_POINT ( 'NONE',  ( 62.90077106633562209, -3.968114999999999615, 8.141649473166729933 ) ) ;
#10501=ORIENTED_EDGE ( 'NONE', *, *, #2002, .F. ) ;
#10526=FACE_OUTER_BOUND ( 'NONE', #5613, .T. ) ;
#10533=LINE ( 'NONE', #14210, #407 ) ;
#10542=AXIS2_PLACEMENT_3D ( 'NONE', #18469, #555, #7075 ) ;
#10556=DIRECTION ( 'NONE',  ( 0.9636276526537417286, 0.000000000000000000, -0.2672484743474500268 ) ) ;
#10557=VERTEX_POINT ( 'NONE', #464 ) ;
#10566=DIRECTION ( 'NONE',  ( 0.000000000000000000, -1.000000000000000000, 0.000000000000000000 ) ) ;
#10578=EDGE_CURVE ( 'NONE', #16397, #16186, #19346, .T. ) ;
#10593=CARTESIAN_POINT ( 'NONE',  ( -17.16618386210371483, -6.903720000000000745, 58.07004290071009223 ) ) ;
#10617=ORIENTED_EDGE ( 'NONE', *, *, #8649, .T. ) ;
#10624=ORIENTED_EDGE ( 'NONE', *, *, #16023, .T. ) ;
#10634=FACE_OUTER_BOUND ( 'NONE', #21786, .T. ) ;
#10644=FACE_OUTER_BOUND ( 'NONE', #16503, .T. ) ;
#10652=AXIS2_PLACEMENT_3D ( 'NONE', #20544, #19228, #10398 ) ;
#10654=DIRECTION ( 'NONE',  ( 0.000000000000000000, 1.000000000000000000, 0.000000000000000000 ) ) ;
#10665=EDGE_LOOP ( 'NONE', ( #20095, #20836, #2811, #11978, #3389, #17198, #20308, #14285, #17873, #8269, #20388, #10617 ) ) ;
#10674=ORIENTED_EDGE ( 'NONE', *, *, #17617, .F. ) ;
#10677=CARTESIAN_POINT ( 'NONE',  ( 10.10534066920194185, -95.96551800000000298, -14.00784516691476966 ) ) ;
#10678=AXIS2_PLACEMENT_3D ( 'NONE', #6172, #969, #19868 ) ;
#10686=ORIENTED_EDGE ( 'NONE', *, *, #12438, .T. ) ;
#10693=VERTEX_POINT ( 'NONE', #785 ) ;
#10697=DIRECTION ( 'NONE',  ( 0.000000000000000000, 1.000000000000000000, 0.000000000000000000 ) ) ;
#10702=LINE ( 'NONE', #17447, #13498 ) ;
#10713=AXIS2_PLACEMENT_3D ( 'NONE', #9380, #1203, #2865 ) ;
#10714=ORIENTED_EDGE ( 'NONE', *, *, #18516, .T. ) ;
#10715=EDGE_CURVE ( 'NONE', #16893, #5161, #20043, .T. ) ;
#10730=DIRECTION ( 'NONE',  ( -0.9964481331860213231, 0.000000000000000000, 0.08420877549337293932 ) ) ;
#10733=ORIENTED_EDGE ( 'NONE', *, *, #6830, .T. ) ;
#10740=DIRECTION ( 'NONE',  ( 0.9685006480810792739, 0.000000000000000000, 0.2490110332224846346 ) ) ;
#10750=VECTOR ( 'NONE', #7617, 1000.000000000000114 ) ;
#10756=CARTESIAN_POINT ( 'NONE',  ( 9.058884679750676128, 128.5105379999999968, -16.32319115207028659 ) ) ;
#10779=ADVANCED_FACE ( 'NONE', ( #17200 ), #15456, .F. ) ;
#10781=UNCERTAINTY_MEASURE_WITH_UNIT (LENGTH_MEASURE( 1.000000000000000082E-05 ), #3721, 'distance_accuracy_value', 'NONE');
#10784=VERTEX_POINT ( 'NONE', #1836 ) ;
#10805=CARTESIAN_POINT ( 'NONE',  ( -18.18961309330695997, -3.266559801243759331, -25.80119252674831998 ) ) ;
#10809=DIRECTION ( 'NONE',  ( -0.6744690509234934073, 0.7360996206939023345, 0.05699866455150641442 ) ) ;
#10813=VERTEX_POINT ( 'NONE', #15351 ) ;
#10824=CARTESIAN_POINT ( 'NONE',  ( 17.10576967688479399, -14.84248999999999974, -11.38708898545455561 ) ) ;
#10826=EDGE_CURVE ( 'NONE', #11404, #21357, #13683, .T. ) ;
#10834=ORIENTED_EDGE ( 'NONE', *, *, #17833, .F. ) ;
#10842=LINE ( 'NONE', #14293, #2501 ) ;
#10848=EDGE_CURVE ( 'NONE', #6259, #14245, #3832, .T. ) ;
#10854=ADVANCED_FACE ( 'NONE', ( #5250 ), #6816, .F. ) ;
#10855=ADVANCED_FACE ( 'NONE', ( #3498 ), #8682, .F. ) ;
#10862=CARTESIAN_POINT ( 'NONE',  ( -16.88621914012359326, 35.81157980123359863, -10.37804376527844141 ) ) ;
#10866=CARTESIAN_POINT ( 'NONE',  ( 9.058884679750676128, 34.52875999999999834, -16.32319115207028659 ) ) ;
#10893=CARTESIAN_POINT ( 'NONE',  ( -19.99570496368815142, 42.13594019876639862, -10.11526441440630286 ) ) ;
#10903=ADVANCED_FACE ( 'NONE', ( #2277 ), #7474, .T. ) ;
#10905=ORIENTED_EDGE ( 'NONE', *, *, #19853, .T. ) ;
#10907=CIRCLE ( 'NONE', #1359, 0.7950200000000000600 ) ;
#10915=LINE ( 'NONE', #2513, #5216 ) ;
#10920=CARTESIAN_POINT ( 'NONE',  ( 31.83819605565793509, -3.968114999999999615, -4.158220719828246814 ) ) ;
#10923=ORIENTED_EDGE ( 'NONE', *, *, #4372, .T. ) ;
#10924=EDGE_LOOP ( 'NONE', ( #21072, #21003, #10155, #12616 ) ) ;
#10929=AXIS2_PLACEMENT_3D ( 'NONE', #21116, #9725, #19576 ) ;
#10940=DIRECTION ( 'NONE',  ( 0.2490110332224846346, 0.000000000000000000, -0.9685006480810792739 ) ) ;
#10948=DIRECTION ( 'NONE',  ( -0.08420877549337300871, 0.000000000000000000, -0.9964481331860212121 ) ) ;
#10956=DIRECTION ( 'NONE',  ( -0.9685006480810794960, 0.000000000000000000, -0.2490110332224836354 ) ) ;
#10959=LINE ( 'NONE', #12631, #2622 ) ;
#10960=DIRECTION ( 'NONE',  ( 0.2490110332224846623, 0.000000000000000000, -0.9685006480810793850 ) ) ;
#10964=VECTOR ( 'NONE', #17272, 1000.000000000000000 ) ;
#10968=AXIS2_PLACEMENT_3D ( 'NONE', #4695, #1581, #19931 ) ;
#10973=EDGE_CURVE ( 'NONE', #2204, #6418, #5597, .T. ) ;
#10983=EDGE_LOOP ( 'NONE', ( #10367, #987, #8490, #3729 ) ) ;
#11003=CARTESIAN_POINT ( 'NONE',  ( 9.256853431388732290, -3.968114999999999615, -17.09316853730597074 ) ) ;
#11013=AXIS2_PLACEMENT_3D ( 'NONE', #3433, #10168, #8503 ) ;
#11017=EDGE_CURVE ( 'NONE', #6939, #7791, #9873, .T. ) ;
#11019=AXIS2_PLACEMENT_3D ( 'NONE', #17239, #7615, #5940 ) ;
#11022=ORIENTED_EDGE ( 'NONE', *, *, #14572, .F. ) ;
#11026=CARTESIAN_POINT ( 'NONE',  ( 10.10534066920194185, -3.968114999999999615, -14.00784516691476966 ) ) ;
#11034=EDGE_LOOP ( 'NONE', ( #889, #7929, #11467, #17458 ) ) ;
#11037=ORIENTED_EDGE ( 'NONE', *, *, #8070, .T. ) ;
#11038=VECTOR ( 'NONE', #2507, 1000.000000000000000 ) ;
#11045=CARTESIAN_POINT ( 'NONE',  ( 46.03750000000000142, 36.51313500000000545, -10.31874999999999964 ) ) ;
#11050=DIRECTION ( 'NONE',  ( 0.9685006480810790519, 0.000000000000000000, 0.2490110332224857170 ) ) ;
#11056=ORIENTED_EDGE ( 'NONE', *, *, #17146, .T. ) ;
#11071=VECTOR ( 'NONE', #11428, 1000.000000000000000 ) ;
#11072=FACE_OUTER_BOUND ( 'NONE', #15555, .T. ) ;
#11074=CARTESIAN_POINT ( 'NONE',  ( 56.47666780297049627, -1.983739999999999393, 1.109116340531466127 ) ) ;
#11079=CARTESIAN_POINT ( 'NONE',  ( 46.03750000000000142, -14.84248999999999974, -10.31874999999999964 ) ) ;
#11084=VERTEX_POINT ( 'NONE', #21611 ) ;
#11099=CIRCLE ( 'NONE', #6507, 1.785937499999999956 ) ;
#11106=ORIENTED_EDGE ( 'NONE', *, *, #19747, .F. ) ;
#11107=CARTESIAN_POINT ( 'NONE',  ( -14.90829243662478909, 34.62011481965967619, -10.03143607188557418 ) ) ;
#11111=ORIENTED_EDGE ( 'NONE', *, *, #8070, .F. ) ;
#11116=LINE ( 'NONE', #10893, #21224 ) ;
#11121=ORIENTED_EDGE ( 'NONE', *, *, #16533, .F. ) ;
#11129=VECTOR ( 'NONE', #6717, 1000.000000000000000 ) ;
#11136=DIRECTION ( 'NONE',  ( 0.000000000000000000, -1.000000000000000000, 0.000000000000000000 ) ) ;
#11138=ORIENTED_EDGE ( 'NONE', *, *, #16446, .T. ) ;
#11141=DIRECTION ( 'NONE',  ( -0.000000000000000000, -1.000000000000000000, 0.000000000000000000 ) ) ;
#11145=ORIENTED_EDGE ( 'NONE', *, *, #7461, .F. ) ;
#11148=EDGE_LOOP ( 'NONE', ( #5877, #19103, #2503, #14349, #14887, #13963, #6694, #4758, #2787, #6455, #17476, #8280, #1638, #8606, #16123, #9531, #4450, #10349, #779, #20739, #13058 ) ) ;
#11151=CARTESIAN_POINT ( 'NONE',  ( -47.86049599909252805, -8.889364999999999739, -23.29373766372935961 ) ) ;
#11153=CARTESIAN_POINT ( 'NONE',  ( -13.97426865170217702, 38.49878000000000355, -10.62412961436650249 ) ) ;
#11159=DIRECTION ( 'NONE',  ( -0.2490110332224836354, 0.000000000000000000, 0.9685006480810794960 ) ) ;
#11167=ORIENTED_EDGE ( 'NONE', *, *, #11524, .F. ) ;
#11172=EDGE_CURVE ( 'NONE', #19449, #14145, #13548, .T. ) ;
#11196=CYLINDRICAL_SURFACE ( 'NONE', #11695, 1.191259999999999319 ) ;
#11198=FACE_OUTER_BOUND ( 'NONE', #14370, .T. ) ;
#11200=EDGE_CURVE ( 'NONE', #7817, #8399, #14092, .T. ) ;
#11203=CARTESIAN_POINT ( 'NONE',  ( 28.56548256563643662, 34.52875999999999834, -12.12873025803960658 ) ) ;
#11225=EDGE_CURVE ( 'NONE', #15795, #15052, #296, .T. ) ;
#11228=VERTEX_POINT ( 'NONE', #1334 ) ;
#11237=VERTEX_POINT ( 'NONE', #11734 ) ;
#11239=CIRCLE ( 'NONE', #10542, 1.785937499999999956 ) ;
#11253=DIRECTION ( 'NONE',  ( 0.000000000000000000, 1.000000000000000000, 0.000000000000000000 ) ) ;
#11256=DIRECTION ( 'NONE',  ( 0.9685006480810794960, 0.000000000000000000, 0.2490110332224836354 ) ) ;
#11259=DIRECTION ( 'NONE',  ( 0.000000000000000000, 1.000000000000000000, 0.000000000000000000 ) ) ;
#11266=ORIENTED_EDGE ( 'NONE', *, *, #11017, .F. ) ;
#11271=ORIENTED_EDGE ( 'NONE', *, *, #2745, .F. ) ;
#11272=EDGE_CURVE ( 'NONE', #12039, #18216, #15169, .T. ) ;
#11280=VECTOR ( 'NONE', #20017, 1000.000000000000114 ) ;
#11286=ORIENTED_EDGE ( 'NONE', *, *, #11430, .T. ) ;
#11291=ORIENTED_EDGE ( 'NONE', *, *, #10578, .F. ) ;
#11297=EDGE_CURVE ( 'NONE', #21613, #16695, #13510, .T. ) ;
#11298=AXIS2_PLACEMENT_3D ( 'NONE', #6530, #21772, #8180 ) ;
#11300=ADVANCED_FACE ( 'NONE', ( #18353 ), #9956, .F. ) ;
#11304=DIRECTION ( 'NONE',  ( -0.9685006480810792739, 0.000000000000000000, -0.2490110332224846346 ) ) ;
#11307=CARTESIAN_POINT ( 'NONE',  ( 30.74535937054756829, 34.52875999999999834, -3.684081112461307317 ) ) ;
#11314=DIRECTION ( 'NONE',  ( 0.000000000000000000, 1.000000000000000000, 0.000000000000000000 ) ) ;
#11322=CARTESIAN_POINT ( 'NONE',  ( 44.28293121686854761, -1.983739999999999393, -31.08068102505560759 ) ) ;
#11327=DIRECTION ( 'NONE',  ( 0.000000000000000000, 1.000000000000000000, 0.000000000000000000 ) ) ;
#11348=ORIENTED_EDGE ( 'NONE', *, *, #4417, .T. ) ;
#11355=AXIS2_PLACEMENT_3D ( 'NONE', #1447, #1660, #6866 ) ;
#11364=ADVANCED_FACE ( 'NONE', ( #3011 ), #4778, .F. ) ;
#11370=VECTOR ( 'NONE', #13707, 1000.000000000000000 ) ;
#11374=DIRECTION ( 'NONE',  ( 0.000000000000000000, 1.000000000000000000, 0.000000000000000000 ) ) ;
#11383=VERTEX_POINT ( 'NONE', #16606 ) ;
#11385=EDGE_CURVE ( 'NONE', #20069, #6991, #11239, .T. ) ;
#11397=ADVANCED_FACE ( 'NONE', ( #3769 ), #8835, .T. ) ;
#11404=VERTEX_POINT ( 'NONE', #19003 ) ;
#11409=ORIENTED_EDGE ( 'NONE', *, *, #20038, .T. ) ;
#11412=VECTOR ( 'NONE', #11964, 1000.000000000000000 ) ;
#11413=EDGE_CURVE ( 'NONE', #17451, #16351, #1761, .T. ) ;
#11417=ORIENTED_EDGE ( 'NONE', *, *, #19561, .T. ) ;
#11428=DIRECTION ( 'NONE',  ( 0.000000000000000000, 1.000000000000000000, 0.000000000000000000 ) ) ;
#11430=EDGE_CURVE ( 'NONE', #21357, #17007, #13751, .T. ) ;
#11440=CARTESIAN_POINT ( 'NONE',  ( 55.81697695389291169, -1.983739999999999393, -11.14520323105768362 ) ) ;
#11442=EDGE_LOOP ( 'NONE', ( #657, #18543, #20759, #6246, #7016 ) ) ;
#11455=ORIENTED_EDGE ( 'NONE', *, *, #2288, .T. ) ;
#11461=AXIS2_PLACEMENT_3D ( 'NONE', #9534, #6217, #4788 ) ;
#11466=AXIS2_PLACEMENT_3D ( 'NONE', #10824, #19110, #3981 ) ;
#11467=ORIENTED_EDGE ( 'NONE', *, *, #4044, .F. ) ;
#11480=DIRECTION ( 'NONE',  ( 0.000000000000000000, 1.000000000000000000, 0.000000000000000000 ) ) ;
#11492=DIRECTION ( 'NONE',  ( 0.000000000000000000, 1.000000000000000000, 0.000000000000000000 ) ) ;
#11493=ORIENTED_EDGE ( 'NONE', *, *, #2745, .T. ) ;
#11499=CARTESIAN_POINT ( 'NONE',  ( 2.915917464538113180, -3.968114999999999615, -18.72348548116188027 ) ) ;
#11502=FACE_OUTER_BOUND ( 'NONE', #9135, .T. ) ;
#11506=CARTESIAN_POINT ( 'NONE',  ( -13.87747867115857936, 36.51313500000000545, -9.458632424640695646 ) ) ;
#11508=CARTESIAN_POINT ( 'NONE',  ( -51.02421882195815783, -8.889364999999999739, -23.02637480153789795 ) ) ;
#11517=EDGE_CURVE ( 'NONE', #17560, #16242, #16793, .T. ) ;
#11518=DIRECTION ( 'NONE',  ( -0.9685006480810794960, 0.000000000000000000, -0.2490110332224836354 ) ) ;
#11520=LINE ( 'NONE', #16511, #10397 ) ;
#11524=EDGE_CURVE ( 'NONE', #11569, #19334, #9926, .T. ) ;
#11533=FACE_OUTER_BOUND ( 'NONE', #11034, .T. ) ;
#11535=ORIENTED_EDGE ( 'NONE', *, *, #15294, .T. ) ;
#11543=VECTOR ( 'NONE', #21270, 1000.000000000000000 ) ;
#11554=ADVANCED_FACE ( 'NONE', ( #9602 ), #10044, .T. ) ;
#11563=DIRECTION ( 'NONE',  ( -0.000000000000000000, -1.000000000000000000, 0.000000000000000000 ) ) ;
#11569=VERTEX_POINT ( 'NONE', #13056 ) ;
#11573=EDGE_LOOP ( 'NONE', ( #13469, #8906, #14471, #18882, #10733, #178, #2971, #19744, #385, #256, #5830, #1532, #8992, #10714, #13195, #5891, #15131, #21649, #6785, #18316, #3177 ) ) ;
#11575=ADVANCED_FACE ( 'NONE', ( #6516 ), #1631, .T. ) ;
#11579=VECTOR ( 'NONE', #2428, 1000.000000000000000 ) ;
#11618=DIRECTION ( 'NONE',  ( -0.2672484743474500268, 0.000000000000000000, -0.9636276526537417286 ) ) ;
#11628=VECTOR ( 'NONE', #4025, 1000.000000000000000 ) ;
#11635=CARTESIAN_POINT ( 'NONE',  ( 29.45491884992628329, -1.983739999999999393, -15.58809351040512325 ) ) ;
#11641=CARTESIAN_POINT ( 'NONE',  ( 19.99312429566830218, -95.96551800000000298, -11.46559883803463720 ) ) ;
#11645=CARTESIAN_POINT ( 'NONE',  ( 20.76310168089343478, -3.968114999999999615, -11.26763008640078212 ) ) ;
#11646=ORIENTED_EDGE ( 'NONE', *, *, #20136, .F. ) ;
#11662=ORIENTED_EDGE ( 'NONE', *, *, #3722, .T. ) ;
#11677=DIRECTION ( 'NONE',  ( 0.000000000000000000, 1.000000000000000000, 0.000000000000000000 ) ) ;
#11686=ORIENTED_EDGE ( 'NONE', *, *, #19187, .T. ) ;
#11688=DIRECTION ( 'NONE',  ( -0.000000000000000000, -1.000000000000000000, 0.000000000000000000 ) ) ;
#11695=AXIS2_PLACEMENT_3D ( 'NONE', #920, #19374, #6320 ) ;
#11699=EDGE_CURVE ( 'NONE', #7796, #17229, #13933, .T. ) ;
#11714=ORIENTED_EDGE ( 'NONE', *, *, #20309, .F. ) ;
#11724=DIRECTION ( 'NONE',  ( 0.2490110332224857170, 0.000000000000000000, -0.9685006480810790519 ) ) ;
#11734=CARTESIAN_POINT ( 'NONE',  ( -46.55710204590916135, 41.43438499999999891, -7.870588902259476605 ) ) ;
#11737=VECTOR ( 'NONE', #6147, 1000.000000000000114 ) ;
#11744=AXIS2_PLACEMENT_3D ( 'NONE', #20734, #5589, #12350 ) ;
#11754=DIRECTION ( 'NONE',  ( 0.000000000000000000, -1.000000000000000000, 0.000000000000000000 ) ) ;
#11756=AXIS2_PLACEMENT_3D ( 'NONE', #13714, #6849, #12042 ) ;
#11768=LINE ( 'NONE', #18494, #4996 ) ;
#11783=EDGE_CURVE ( 'NONE', #20277, #21616, #13481, .T. ) ;
#11786=AXIS2_PLACEMENT_3D ( 'NONE', #17203, #3728, #179 ) ;
#11800=ORIENTED_EDGE ( 'NONE', *, *, #2950, .F. ) ;
#11802=DIRECTION ( 'NONE',  ( -0.08420877549337300871, 0.000000000000000000, -0.9964481331860212121 ) ) ;
#11810=CARTESIAN_POINT ( 'NONE',  ( -14.39647200192898779, -1.983739999999848624, -9.747027169376975664 ) ) ;
#11812=LINE ( 'NONE', #3404, #16449 ) ;
#11814=ORIENTED_EDGE ( 'NONE', *, *, #15294, .F. ) ;
#11826=ORIENTED_EDGE ( 'NONE', *, *, #14416, .T. ) ;
#11828=CARTESIAN_POINT ( 'NONE',  ( 12.79472653632228507, -1.983739999999999393, -13.31637763425449883 ) ) ;
#11832=LINE ( 'NONE', #2306, #4234 ) ;
#11833=EDGE_CURVE ( 'NONE', #20277, #3371, #17983, .T. ) ;
#11835=CARTESIAN_POINT ( 'NONE',  ( 3.360635606688116894, 36.51313500000000545, -20.45316710734507026 ) ) ;
#11843=VECTOR ( 'NONE', #12244, 1000.000000000000000 ) ;
#11852=EDGE_CURVE ( 'NONE', #15164, #15141, #11965, .T. ) ;
#11855=EDGE_CURVE ( 'NONE', #17362, #19935, #18760, .T. ) ;
#11862=CARTESIAN_POINT ( 'NONE',  ( 46.03750000000000142, -3.968114999999999615, -10.31874999999999964 ) ) ;
#11867=ORIENTED_EDGE ( 'NONE', *, *, #2107, .T. ) ;
#11871=FACE_OUTER_BOUND ( 'NONE', #10382, .T. ) ;
#11874=CARTESIAN_POINT ( 'NONE',  ( 29.45491884992628329, 34.52875999999999834, -15.58809351040512325 ) ) ;
#11876=DIRECTION ( 'NONE',  ( -0.000000000000000000, -1.000000000000000000, 0.000000000000000000 ) ) ;
#11882=EDGE_LOOP ( 'NONE', ( #7027, #13233, #740, #1339, #7201, #2147, #6157, #16795, #16772, #4779, #20930, #18671 ) ) ;
#11891=VERTEX_POINT ( 'NONE', #15916 ) ;
#11894=ORIENTED_EDGE ( 'NONE', *, *, #13068, .T. ) ;
#11900=ORIENTED_EDGE ( 'NONE', *, *, #11272, .T. ) ;
#11904=ORIENTED_EDGE ( 'NONE', *, *, #4044, .T. ) ;
#11905=CARTESIAN_POINT ( 'NONE',  ( -24.21104940531825633, 43.41875999999999891, -25.29232732678598339 ) ) ;
#11919=EDGE_LOOP ( 'NONE', ( #19096, #5827, #8924, #1310, #16483 ) ) ;
#11934=PLANE ( 'NONE',  #15735 ) ;
#11943=EDGE_CURVE ( 'NONE', #9466, #16242, #10210, .T. ) ;
#11945=ORIENTED_EDGE ( 'NONE', *, *, #19853, .F. ) ;
#11949=ORIENTED_EDGE ( 'NONE', *, *, #3020, .F. ) ;
#11954=CARTESIAN_POINT ( 'NONE',  ( 59.61686353177688602, -3.968114999999999615, -0.7993558564620834028 ) ) ;
#11964=DIRECTION ( 'NONE',  ( 0.08420877549337300871, 0.000000000000000000, 0.9964481331860212121 ) ) ;
#11965=CIRCLE ( 'NONE', #16231, 1.191259999999998209 ) ;
#11974=ADVANCED_FACE ( 'NONE', ( #4042 ), #17752, .F. ) ;
#11977=VECTOR ( 'NONE', #12876, 1000.000000000000000 ) ;
#11978=ORIENTED_EDGE ( 'NONE', *, *, #7088, .T. ) ;
#11985=CARTESIAN_POINT ( 'NONE',  ( 46.03750000000000142, -1.983739999999999393, -10.31874999999999964 ) ) ;
#12014=VERTEX_POINT ( 'NONE', #16002 ) ;
#12019=LINE ( 'NONE', #7034, #20644 ) ;
#12021=ADVANCED_FACE ( 'NONE', ( #17302 ), #7680, .F. ) ;
#12023=ORIENTED_EDGE ( 'NONE', *, *, #6278, .T. ) ;
#12026=DIRECTION ( 'NONE',  ( 0.000000000000000000, 1.000000000000000000, 0.000000000000000000 ) ) ;
#12027=CARTESIAN_POINT ( 'NONE',  ( 30.74535937054756829, -3.968114999999999615, -3.684081112461307317 ) ) ;
#12039=VERTEX_POINT ( 'NONE', #17532 ) ;
#12040=CIRCLE ( 'NONE', #14889, 0.7950200000000000600 ) ;
#12042=DIRECTION ( 'NONE',  ( 0.9964481331860212121, 0.000000000000000000, -0.08420877549337300871 ) ) ;
#12043=ORIENTED_EDGE ( 'NONE', *, *, #3422, .F. ) ;
#12049=CARTESIAN_POINT ( 'NONE',  ( 28.56548256563643662, -14.84248999999999974, -12.12873025803960658 ) ) ;
#12051=EDGE_CURVE ( 'NONE', #6063, #9888, #3933, .T. ) ;
#12062=CARTESIAN_POINT ( 'NONE',  ( 3.805353748838121053, 34.52875999999999834, -22.18284873352824960 ) ) ;
#12064=EDGE_LOOP ( 'NONE', ( #13007, #957, #11867, #7076 ) ) ;
#12068=AXIS2_PLACEMENT_3D ( 'NONE', #5523, #20664, #13847 ) ;
#12076=ADVANCED_FACE ( 'NONE', ( #6012 ), #7254, .F. ) ;
#12082=MECHANICAL_DESIGN_GEOMETRIC_PRESENTATION_REPRESENTATION('',(#2139),#7487);
#12084=VECTOR ( 'NONE', #17340, 1000.000000000000000 ) ;
#12090=LINE ( 'NONE', #358, #6746 ) ;
#12091=VECTOR ( 'NONE', #7168, 1000.000000000000114 ) ;
#12096=CYLINDRICAL_SURFACE ( 'NONE', #6752, 1.191259999999999986 ) ;
#12101=ORIENTED_EDGE ( 'NONE', *, *, #19262, .F. ) ;
#12103=DIRECTION ( 'NONE',  ( 0.000000000000000000, -1.000000000000000000, 0.000000000000000000 ) ) ;
#12107=AXIS2_PLACEMENT_3D ( 'NONE', #11440, #21269, #3037 ) ;
#12130=DIRECTION ( 'NONE',  ( 0.2490110332224857170, 0.000000000000000000, -0.9685006480810790519 ) ) ;
#12137=ORIENTED_EDGE ( 'NONE', *, *, #18200, .T. ) ;
#12144=DIRECTION ( 'NONE',  ( 0.000000000000000000, 1.000000000000000000, 0.000000000000000000 ) ) ;
#12146=LINE ( 'NONE', #13809, #9902 ) ;
#12148=DIRECTION ( 'NONE',  ( 0.000000000000000000, 1.000000000000000000, 0.000000000000000000 ) ) ;
#12152=ORIENTED_EDGE ( 'NONE', *, *, #14024, .T. ) ;
#12157=EDGE_LOOP ( 'NONE', ( #9356, #7934, #9920, #2763 ) ) ;
#12158=VERTEX_POINT ( 'NONE', #9661 ) ;
#12171=VECTOR ( 'NONE', #18584, 1000.000000000000000 ) ;
#12174=DIRECTION ( 'NONE',  ( -0.2490110332224848011, 0.000000000000000000, 0.9685006480810792739 ) ) ;
#12203=EDGE_CURVE ( 'NONE', #18449, #6418, #7895, .T. ) ;
#12211=EDGE_CURVE ( 'NONE', #1715, #3845, #7665, .T. ) ;
#12213=EDGE_CURVE ( 'NONE', #10171, #9714, #9409, .T. ) ;
#12221=DIRECTION ( 'NONE',  ( 0.2490110332224846346, 0.000000000000000000, -0.9685006480810792739 ) ) ;
#12230=DIRECTION ( 'NONE',  ( 0.000000000000000000, 1.000000000000000000, 0.000000000000000000 ) ) ;
#12235=ADVANCED_FACE ( 'NONE', ( #1259 ), #9863, .F. ) ;
#12243=LINE ( 'NONE', #6824, #2826 ) ;
#12244=DIRECTION ( 'NONE',  ( 0.9636276526537417286, 0.000000000000000000, -0.2672484743474500268 ) ) ;
#12248=CARTESIAN_POINT ( 'NONE',  ( -13.87747867115857936, -3.968114999999999615, -9.458632424640695646 ) ) ;
#12253=ORIENTED_EDGE ( 'NONE', *, *, #17748, .T. ) ;
#12260=ORIENTED_EDGE ( 'NONE', *, *, #19488, .T. ) ;
#12264=CIRCLE ( 'NONE', #13686, 9.524999999999996803 ) ;
#12265=VERTEX_POINT ( 'NONE', #2814 ) ;
#12267=ORIENTED_EDGE ( 'NONE', *, *, #7931, .F. ) ;
#12270=PLANE ( 'NONE',  #11466 ) ;
#12272=CARTESIAN_POINT ( 'NONE',  ( 17.79723720954694954, 36.51313500000000545, -14.07647485258271303 ) ) ;
#12278=DIRECTION ( 'NONE',  ( 0.000000000000000000, 1.000000000000000000, 0.000000000000000000 ) ) ;
#12280=ADVANCED_FACE ( 'NONE', ( #3038 ), #9762, .F. ) ;
#12293=CARTESIAN_POINT ( 'NONE',  ( -21.29909891687151813, -9.590920198756240467, -25.53841317587618320 ) ) ;
#12303=DIRECTION ( 'NONE',  ( 0.2490110332224848289, 0.000000000000000000, -0.9685006480810792739 ) ) ;
#12313=CARTESIAN_POINT ( 'NONE',  ( 44.28293121686854761, 34.52875999999999834, -31.08068102505560759 ) ) ;
#12330=EDGE_CURVE ( 'NONE', #7937, #19449, #6500, .T. ) ;
#12340=ORIENTED_EDGE ( 'NONE', *, *, #15793, .F. ) ;
#12345=CARTESIAN_POINT ( 'NONE',  ( 12.79472653632228507, -3.968114999999999615, -13.31637763425449883 ) ) ;
#12350=DIRECTION ( 'NONE',  ( -0.9964481331860212121, 0.000000000000000000, 0.08420877549337293932 ) ) ;
#12354=CARTESIAN_POINT ( 'NONE',  ( 13.28822531734660828, -1.983739999999999393, -15.23578611614444078 ) ) ;
#12363=CARTESIAN_POINT ( 'NONE',  ( 22.22454659879084460, -1.983739999999999393, -13.75904720189594244 ) ) ;
#12372=ADVANCED_FACE ( 'NONE', ( #11871 ), #10095, .T. ) ;
#12377=ORIENTED_EDGE ( 'NONE', *, *, #18142, .F. ) ;
#12378=CIRCLE ( 'NONE', #352, 0.7950200000000000600 ) ;
#12383=DIRECTION ( 'NONE',  ( -0.000000000000000000, -1.000000000000000000, 0.000000000000000000 ) ) ;
#12386=FACE_OUTER_BOUND ( 'NONE', #4639, .T. ) ;
#12391=CARTESIAN_POINT ( 'NONE',  ( 12.79472653632228507, 34.52875999999999834, -13.31637763425449883 ) ) ;
#12395=VERTEX_POINT ( 'NONE', #6888 ) ;
#12398=FACE_OUTER_BOUND ( 'NONE', #13836, .T. ) ;
#12403=DIRECTION ( 'NONE',  ( -0.000000000000000000, -1.000000000000000000, 0.000000000000000000 ) ) ;
#12409=VECTOR ( 'NONE', #12539, 1000.000000000000000 ) ;
#12410=CIRCLE ( 'NONE', #19778, 5.158739999999998105 ) ;
#12428=VECTOR ( 'NONE', #8295, 1000.000000000000000 ) ;
#12437=AXIS2_PLACEMENT_3D ( 'NONE', #19322, #8939, #5620 ) ;
#12438=EDGE_CURVE ( 'NONE', #17007, #17560, #18818, .T. ) ;
#12441=ORIENTED_EDGE ( 'NONE', *, *, #2518, .F. ) ;
#12444=CARTESIAN_POINT ( 'NONE',  ( 9.907371917564091746, -1.983739999999999393, -13.23786778167655243 ) ) ;
#12446=CIRCLE ( 'NONE', #14227, 1.785937499999999956 ) ;
#12455=ORIENTED_EDGE ( 'NONE', *, *, #17236, .F. ) ;
#12463=CIRCLE ( 'NONE', #2924, 0.3962399999999998701 ) ;
#12465=VERTEX_POINT ( 'NONE', #1098 ) ;
#12470=CARTESIAN_POINT ( 'NONE',  ( 21.25660046192028929, -1.983739999999999393, -13.18703856829094079 ) ) ;
#12475=CARTESIAN_POINT ( 'NONE',  ( 46.03750000000000142, 34.52875999999999834, -10.31874999999999964 ) ) ;
#12478=DIRECTION ( 'NONE',  ( 0.6744690509234938514, -0.7360996206939018904, -0.05699866455150646993 ) ) ;
#12483=ORIENTED_EDGE ( 'NONE', *, *, #19071, .T. ) ;
#12493=EDGE_CURVE ( 'NONE', #20833, #21044, #21104, .T. ) ;
#12496=VECTOR ( 'NONE', #10809, 1000.000000000000114 ) ;
#12500=DIRECTION ( 'NONE',  ( 0.000000000000000000, 1.000000000000000000, 0.000000000000000000 ) ) ;
#12523=EDGE_CURVE ( 'NONE', #7062, #17451, #7627, .T. ) ;
#12524=CYLINDRICAL_SURFACE ( 'NONE', #15327, 3.970020000000000326 ) ;
#12528=CARTESIAN_POINT ( 'NONE',  ( 21.25660046192028929, -3.968114999999999615, -13.18703856829094079 ) ) ;
#12533=FACE_OUTER_BOUND ( 'NONE', #12595, .T. ) ;
#12534=CYLINDRICAL_SURFACE ( 'NONE', #17724, 0.7950200000000000600 ) ;
#12538=CARTESIAN_POINT ( 'NONE',  ( -16.07247711516169275, -2.588178535606159958, -10.44681224123558039 ) ) ;
#12539=DIRECTION ( 'NONE',  ( 0.000000000000000000, 1.000000000000000000, 0.000000000000000000 ) ) ;
#12541=ORIENTED_EDGE ( 'NONE', *, *, #20170, .F. ) ;
#12543=DIRECTION ( 'NONE',  ( -0.2490110332224846623, 0.000000000000000000, 0.9685006480810793850 ) ) ;
#12544=EDGE_CURVE ( 'NONE', #2636, #12014, #1297, .T. ) ;
#12547=LINE ( 'NONE', #7439, #11977 ) ;
#12560=CARTESIAN_POINT ( 'NONE',  ( -47.86049599909252805, 41.43438499999999891, -23.29373766372935961 ) ) ;
#12564=AXIS2_PLACEMENT_3D ( 'NONE', #11153, #972, #4745 ) ;
#12566=ADVANCED_FACE ( 'NONE', ( #5756 ), #16268, .T. ) ;
#12582=CARTESIAN_POINT ( 'NONE',  ( 55.81697695389291169, -14.84248999999999974, -11.14520323105768362 ) ) ;
#12584=LINE ( 'NONE', #19202, #12856 ) ;
#12586=CYLINDRICAL_SURFACE ( 'NONE', #12646, 15.47812499999999680 ) ;
#12588=VERTEX_POINT ( 'NONE', #20886 ) ;
#12589=EDGE_CURVE ( 'NONE', #16799, #14245, #12954, .T. ) ;
#12595=EDGE_LOOP ( 'NONE', ( #9040, #19911, #6660, #11409 ) ) ;
#12599=DIRECTION ( 'NONE',  ( -0.08420877549337300871, 0.000000000000000000, -0.9964481331860212121 ) ) ;
#12613=DIRECTION ( 'NONE',  ( 0.000000000000000000, 1.000000000000000000, 0.000000000000000000 ) ) ;
#12616=ORIENTED_EDGE ( 'NONE', *, *, #20013, .T. ) ;
#12625=LINE ( 'NONE', #6382, #1178 ) ;
#12629=ADVANCED_FACE ( 'NONE', ( #13487 ), #7954, .T. ) ;
#12631=CARTESIAN_POINT ( 'NONE',  ( -18.18961309330695997, 35.81157980123359863, -25.80119252674831998 ) ) ;
#12646=AXIS2_PLACEMENT_3D ( 'NONE', #21182, #17448, #2407 ) ;
#12648=VERTEX_POINT ( 'NONE', #3317 ) ;
#12667=EDGE_LOOP ( 'NONE', ( #1490, #1367, #16084, #20304 ) ) ;
#12684=EDGE_CURVE ( 'NONE', #1375, #4259, #16587, .T. ) ;
#12695=DIRECTION ( 'NONE',  ( 0.9964481331860212121, 0.000000000000000000, -0.08420877549337300871 ) ) ;
#12704=VECTOR ( 'NONE', #17713, 1000.000000000000000 ) ;
#12705=LINE ( 'NONE', #2422, #9957 ) ;
#12708=LINE ( 'NONE', #2860, #10750 ) ;
#12713=CARTESIAN_POINT ( 'NONE',  ( 9.058884679750676128, -1.983739999999999393, -16.32319115207028659 ) ) ;
#12715=CARTESIAN_POINT ( 'NONE',  ( 10.10534066920194185, -1.983739999999999393, -14.00784516691476966 ) ) ;
#12724=ORIENTED_EDGE ( 'NONE', *, *, #20453, .F. ) ;
#12762=CIRCLE ( 'NONE', #8495, 20.83593750000000000 ) ;
#12763=ORIENTED_EDGE ( 'NONE', *, *, #12544, .F. ) ;
#12769=ORIENTED_EDGE ( 'NONE', *, *, #9353, .T. ) ;
#12774=CARTESIAN_POINT ( 'NONE',  ( 46.03750000000000142, -3.968114999999999615, -10.31874999999999964 ) ) ;
#12784=VECTOR ( 'NONE', #84, 1000.000000000000000 ) ;
#12787=CARTESIAN_POINT ( 'NONE',  ( 1.581041518826207248, -3.968114999999999615, -20.30277549736237575 ) ) ;
#12791=CARTESIAN_POINT ( 'NONE',  ( 30.42699695299585017, 34.52875999999999834, -4.832012189960551041 ) ) ;
#12792=ORIENTED_EDGE ( 'NONE', *, *, #20360, .F. ) ;
#12803=VECTOR ( 'NONE', #1985, 1000.000000000000000 ) ;
#12811=EDGE_LOOP ( 'NONE', ( #12769, #18787, #9256, #443 ) ) ;
#12817=EDGE_LOOP ( 'NONE', ( #16435, #3442, #6517, #5387 ) ) ;
#12827=VECTOR ( 'NONE', #13110, 1000.000000000000000 ) ;
#12829=CYLINDRICAL_SURFACE ( 'NONE', #17738, 1.983739999999995618 ) ;
#12834=ORIENTED_EDGE ( 'NONE', *, *, #5765, .F. ) ;
#12838=CARTESIAN_POINT ( 'NONE',  ( 46.03750000000000142, 36.51313500000000545, -10.31874999999999964 ) ) ;
#12840=ORIENTED_EDGE ( 'NONE', *, *, #2080, .F. ) ;
#12843=CARTESIAN_POINT ( 'NONE',  ( 21.25660046192028929, 36.51313500000000545, -13.18703856829094079 ) ) ;
#12856=VECTOR ( 'NONE', #20628, 1000.000000000000114 ) ;
#12858=DIRECTION ( 'NONE',  ( 0.000000000000000000, -1.000000000000000000, 0.000000000000000000 ) ) ;
#12868=EDGE_LOOP ( 'NONE', ( #9368, #12377, #2305, #21724 ) ) ;
#12871=ORIENTED_EDGE ( 'NONE', *, *, #14923, .F. ) ;
#12876=DIRECTION ( 'NONE',  ( 0.08420877549337300871, 0.000000000000000000, 0.9964481331860212121 ) ) ;
#12884=LINE ( 'NONE', #11203, #11071 ) ;
#12907=CIRCLE ( 'NONE', #5825, 1.785937499999998179 ) ;
#12922=CARTESIAN_POINT ( 'NONE',  ( 55.52866846859685523, -14.84248999999999974, -11.12083858657437752 ) ) ;
#12928=LINE ( 'NONE', #10920, #4966 ) ;
#12933=AXIS2_PLACEMENT_3D ( 'NONE', #19029, #16936, #18700 ) ;
#12954=LINE ( 'NONE', #19662, #8348 ) ;
#12975=ORIENTED_EDGE ( 'NONE', *, *, #18264, .F. ) ;
#13002=ORIENTED_EDGE ( 'NONE', *, *, #14127, .T. ) ;
#13006=ADVANCED_BREP_SHAPE_REPRESENTATION ( '', ( #5939, #2234 ), #3303 ) ;
#13007=ORIENTED_EDGE ( 'NONE', *, *, #19891, .F. ) ;
#13018=ORIENTED_EDGE ( 'NONE', *, *, #13043, .T. ) ;
#13020=CARTESIAN_POINT ( 'NONE',  ( 19.99312429566830218, -3.968114999999999615, -11.46559883803463720 ) ) ;
#13028=DIRECTION ( 'NONE',  ( -0.9685006480810794960, 0.000000000000000000, -0.2490110332224836354 ) ) ;
#13041=VERTEX_POINT ( 'NONE', #853 ) ;
#13043=EDGE_CURVE ( 'NONE', #11383, #4031, #19408, .T. ) ;
#13045=DIRECTION ( 'NONE',  ( 0.000000000000000000, 1.000000000000000000, 0.000000000000000000 ) ) ;
#13054=DIRECTION ( 'NONE',  ( 0.000000000000000000, 1.000000000000000000, 0.000000000000000000 ) ) ;
#13056=CARTESIAN_POINT ( 'NONE',  ( -15.39353573898878658, -4.587157632697119958, -10.30107656633069979 ) ) ;
#13058=ORIENTED_EDGE ( 'NONE', *, *, #2345, .F. ) ;
#13063=ORIENTED_EDGE ( 'NONE', *, *, #6830, .F. ) ;
#13068=EDGE_CURVE ( 'NONE', #3226, #6728, #12264, .T. ) ;
#13069=CIRCLE ( 'NONE', #2463, 1.785937499999998179 ) ;
#13081=CYLINDRICAL_SURFACE ( 'NONE', #8175, 0.7950200000000000600 ) ;
#13091=DIRECTION ( 'NONE',  ( 0.2490110332224846346, 0.000000000000000000, -0.9685006480810792739 ) ) ;
#13095=ADVANCED_FACE ( 'NONE', ( #627 ), #17554, .T. ) ;
#13107=FACE_BOUND ( 'NONE', #18500, .T. ) ;
#13108=VECTOR ( 'NONE', #17646, 1000.000000000000000 ) ;
#13110=DIRECTION ( 'NONE',  ( -0.08420877549337300871, 0.000000000000000000, -0.9964481331860212121 ) ) ;
#13115=DIRECTION ( 'NONE',  ( 0.2490110332224846623, 0.000000000000000000, -0.9685006480810793850 ) ) ;
#13150=CIRCLE ( 'NONE', #1109, 0.7950200000000003930 ) ;
#13154=VECTOR ( 'NONE', #9273, 1000.000000000000114 ) ;
#13156=CARTESIAN_POINT ( 'NONE',  ( 19.79515554403045741, 34.52875999999999834, -10.69562145279641996 ) ) ;
#13157=LINE ( 'NONE', #11151, #18164 ) ;
#13158=DIRECTION ( 'NONE',  ( 0.08420877549337300871, 0.000000000000000000, 0.9964481331860212121 ) ) ;
#13161=AXIS2_PLACEMENT_3D ( 'NONE', #11641, #20026, #2808 ) ;
#13163=LINE ( 'NONE', #4749, #8933 ) ;
#13171=( BOUNDED_CURVE ( )  B_SPLINE_CURVE ( 3, ( #5158, #3506, #15363, #8267 ),
 .UNSPECIFIED., .F., .F. ) 
 B_SPLINE_CURVE_WITH_KNOTS ( ( 4, 4 ),
 ( 4.712388980381386538, 5.283302931178984529 ),
 .UNSPECIFIED. ) 
 CURVE ( )  GEOMETRIC_REPRESENTATION_ITEM ( )  RATIONAL_B_SPLINE_CURVE ( ( 1.000000000000000000, 0.9730220469480294065, 0.9730220469480294065, 1.000000000000000000 ) ) 
 REPRESENTATION_ITEM ( '' )  );
#13178=EDGE_CURVE ( 'NONE', #6430, #5334, #9355, .T. ) ;
#13184=DIRECTION ( 'NONE',  ( 0.000000000000000000, 1.000000000000000000, 0.000000000000000000 ) ) ;
#13194=CARTESIAN_POINT ( 'NONE',  ( 17.87574706213523612, 34.52875999999999834, -11.18912023382283571 ) ) ;
#13195=ORIENTED_EDGE ( 'NONE', *, *, #9250, .T. ) ;
#13206=AXIS2_PLACEMENT_3D ( 'NONE', #16451, #7921, #19732 ) ;
#13207=CARTESIAN_POINT ( 'NONE',  ( -22.75431282566211522, 40.79338547039380103, -25.41543459098148716 ) ) ;
#13217=EDGE_CURVE ( 'NONE', #12039, #1153, #13793, .T. ) ;
#13220=PLANE ( 'NONE',  #10968 ) ;
#13223=CARTESIAN_POINT ( 'NONE',  ( -22.90765545213488963, 43.41875999999999891, -9.869178565316103047 ) ) ;
#13233=ORIENTED_EDGE ( 'NONE', *, *, #5156, .F. ) ;
#13244=AXIS2_PLACEMENT_3D ( 'NONE', #698, #8990, #5890 ) ;
#13248=ORIENTED_EDGE ( 'NONE', *, *, #11783, .T. ) ;
#13255=DIRECTION ( 'NONE',  ( 0.2490110332224846623, 0.000000000000000000, -0.9685006480810793850 ) ) ;
#13258=ORIENTED_EDGE ( 'NONE', *, *, #1657, .F. ) ;
#13260=ORIENTED_EDGE ( 'NONE', *, *, #1953, .T. ) ;
#13265=ORIENTED_EDGE ( 'NONE', *, *, #2472, .T. ) ;
#13273=ORIENTED_EDGE ( 'NONE', *, *, #19071, .F. ) ;
#13284=ORIENTED_EDGE ( 'NONE', *, *, #1564, .F. ) ;
#13286=ORIENTED_EDGE ( 'NONE', *, *, #5349, .T. ) ;
#13296=DIRECTION ( 'NONE',  ( -0.9964481331860213231, 0.000000000000000000, 0.08420877549337203727 ) ) ;
#13298=ORIENTED_EDGE ( 'NONE', *, *, #8686, .T. ) ;
#13309=LINE ( 'NONE', #4561, #2451 ) ;
#13316=LINE ( 'NONE', #18370, #21518 ) ;
#13317=DIRECTION ( 'NONE',  ( -0.000000000000000000, -1.000000000000000000, 0.000000000000000000 ) ) ;
#13324=CARTESIAN_POINT ( 'NONE',  ( -24.20935654380574320, -8.889364999999999739, -25.29247038871795894 ) ) ;
#13338=CARTESIAN_POINT ( 'NONE',  ( 14.05820270259704152, -1.983739999999999393, -15.03781736451272444 ) ) ;
#13364=EDGE_CURVE ( 'NONE', #9466, #20607, #3708, .T. ) ;
#13376=CARTESIAN_POINT ( 'NONE',  ( 9.828862065001116477, -1.983739999999999393, -16.12522240043857025 ) ) ;
#13378=VERTEX_POINT ( 'NONE', #13560 ) ;
#13381=ORIENTED_EDGE ( 'NONE', *, *, #11385, .T. ) ;
#13425=CARTESIAN_POINT ( 'NONE',  ( -15.61825442841409384, -4.819421976693936571, -10.42024638159965555 ) ) ;
#13438=EDGE_CURVE ( 'NONE', #17882, #2409, #20485, .T. ) ;
#13450=EDGE_LOOP ( 'NONE', ( #5372, #21841, #8250, #7149 ) ) ;
#13458=PLANE ( 'NONE',  #20844 ) ;
#13462=ORIENTED_EDGE ( 'NONE', *, *, #21733, .T. ) ;
#13466=EDGE_LOOP ( 'NONE', ( #13286, #8072, #11535, #6191 ) ) ;
#13467=CIRCLE ( 'NONE', #20133, 0.7950200000000003930 ) ;
#13469=ORIENTED_EDGE ( 'NONE', *, *, #12211, .T. ) ;
#13470=DIRECTION ( 'NONE',  ( 0.000000000000000000, 1.000000000000000000, 0.000000000000000000 ) ) ;
#13479=EDGE_CURVE ( 'NONE', #9714, #21739, #18841, .T. ) ;
#13480=CARTESIAN_POINT ( 'NONE',  ( 9.907371917564091746, -3.968114999999999615, -13.23786778167655243 ) ) ;
#13481=LINE ( 'NONE', #20631, #18660 ) ;
#13482=VERTEX_POINT ( 'NONE', #17187 ) ;
#13484=ORIENTED_EDGE ( 'NONE', *, *, #336, .F. ) ;
#13485=VECTOR ( 'NONE', #17577, 1000.000000000000000 ) ;
#13487=FACE_OUTER_BOUND ( 'NONE', #13466, .T. ) ;
#13488=EDGE_LOOP ( 'NONE', ( #6844, #13284, #18767, #18090, #15928 ) ) ;
#13489=ORIENTED_EDGE ( 'NONE', *, *, #20842, .F. ) ;
#13493=CARTESIAN_POINT ( 'NONE',  ( -15.27766260488554195, -5.953760000000000829, -26.04727837583638461 ) ) ;
#13495=VECTOR ( 'NONE', #14640, 1000.000000000000000 ) ;
#13498=VECTOR ( 'NONE', #15802, 1000.000000000000000 ) ;
#13500=DIRECTION ( 'NONE',  ( -0.2490110332224846346, 0.000000000000000000, 0.9685006480810792739 ) ) ;
#13504=CARTESIAN_POINT ( 'NONE',  ( -19.99570496368815142, -9.590920198756240467, -10.11526441440630286 ) ) ;
#13505=ORIENTED_EDGE ( 'NONE', *, *, #16187, .T. ) ;
#13510=LINE ( 'NONE', #13194, #19366 ) ;
#13514=COLOUR_RGB ( '', 0.66274510, 0.83137255, 0.94901961) ;
#13516=LINE ( 'NONE', #12062, #5342 ) ;
#13519=VECTOR ( 'NONE', #4805, 1000.000000000000000 ) ;
#13529=LINE ( 'NONE', #5209, #11412 ) ;
#13540=CARTESIAN_POINT ( 'NONE',  ( -15.84345693979051894, -5.059254600095735022, -10.46616649349276074 ) ) ;
#13545=CARTESIAN_POINT ( 'NONE',  ( 3.805353748838121053, -3.968114999999999615, -22.18284873352824960 ) ) ;
#13548=LINE ( 'NONE', #7001, #17609 ) ;
#13550=CARTESIAN_POINT ( 'NONE',  ( -24.20935654380574320, 41.43438499999999891, -25.29247038871795894 ) ) ;
#13560=CARTESIAN_POINT ( 'NONE',  ( 9.828862065001116477, 34.52875999999999834, -16.12522240043857025 ) ) ;
#13562=ORIENTED_EDGE ( 'NONE', *, *, #11297, .T. ) ;
#13580=ORIENTED_EDGE ( 'NONE', *, *, #9353, .F. ) ;
#13581=CIRCLE ( 'NONE', #14656, 9.524999999999996803 ) ;
#13587=CARTESIAN_POINT ( 'NONE',  ( 66.79943102505561114, -3.968114999999999615, -12.07331878313145168 ) ) ;
#13604=ORIENTED_EDGE ( 'NONE', *, *, #20038, .F. ) ;
#13614=CARTESIAN_POINT ( 'NONE',  ( 11.42842559562532578, 36.51313500000000545, 1.673196738795719174 ) ) ;
#13615=DIRECTION ( 'NONE',  ( 0.2490110332224846623, 0.000000000000000000, -0.9685006480810793850 ) ) ;
#13634=CARTESIAN_POINT ( 'NONE',  ( -46.55773479047372376, 43.41875999999999891, -7.870535429687039120 ) ) ;
#13644=CARTESIAN_POINT ( 'NONE',  ( 17.02725982432203367, 36.51313500000000545, -14.27444360421403857 ) ) ;
#13659=DIRECTION ( 'NONE',  ( 0.000000000000000000, 1.000000000000000000, 0.000000000000000000 ) ) ;
#13681=VERTEX_POINT ( 'NONE', #9331 ) ;
#13683=LINE ( 'NONE', #20279, #2410 ) ;
#13685=EDGE_CURVE ( 'NONE', #18743, #16186, #5689, .T. ) ;
#13686=AXIS2_PLACEMENT_3D ( 'NONE', #12475, #2508, #19529 ) ;
#13702=VERTEX_POINT ( 'NONE', #4367 ) ;
#13707=DIRECTION ( 'NONE',  ( -0.000000000000000000, -1.000000000000000000, 0.000000000000000000 ) ) ;
#13708=EDGE_LOOP ( 'NONE', ( #15266, #11714, #12792, #6489 ) ) ;
#13714=CARTESIAN_POINT ( 'NONE',  ( 46.03750000000000142, -3.968114999999999615, -10.31874999999999964 ) ) ;
#13715=ADVANCED_FACE ( 'NONE', ( #14548 ), #4037, .F. ) ;
#13723=FACE_OUTER_BOUND ( 'NONE', #10924, .T. ) ;
#13726=CARTESIAN_POINT ( 'NONE',  ( -49.72082486877479113, -5.714364999999999029, -7.603226040068017610 ) ) ;
#13731=FACE_OUTER_BOUND ( 'NONE', #4815, .T. ) ;
#13734=EDGE_CURVE ( 'NONE', #2204, #6613, #1354, .T. ) ;
#13744=DIRECTION ( 'NONE',  ( -0.08420877549337300871, 0.000000000000000000, -0.9964481331860212121 ) ) ;
#13751=CIRCLE ( 'NONE', #4555, 0.7950200000000000600 ) ;
#13757=FACE_OUTER_BOUND ( 'NONE', #19985, .T. ) ;
#13762=ADVANCED_FACE ( 'NONE', ( #19820 ), #13220, .T. ) ;
#13777=FACE_OUTER_BOUND ( 'NONE', #15818, .T. ) ;
#13786=CARTESIAN_POINT ( 'NONE',  ( 13.28822531734660828, 34.52875999999999834, -15.23578611614444078 ) ) ;
#13793=CIRCLE ( 'NONE', #19412, 0.3962400000000000366 ) ;
#13798=DIRECTION ( 'NONE',  ( 0.08420877549337300871, 0.000000000000000000, 0.9964481331860212121 ) ) ;
#13807=DIRECTION ( 'NONE',  ( -0.08420877549337300871, 0.000000000000000000, -0.9964481331860212121 ) ) ;
#13808=CYLINDRICAL_SURFACE ( 'NONE', #2184, 9.524999999999996803 ) ;
#13809=CARTESIAN_POINT ( 'NONE',  ( 1.581041518826207692, -14.84248999999999974, -20.30277549736237575 ) ) ;
#13810=CARTESIAN_POINT ( 'NONE',  ( 20.76310168089343478, -1.983739999999999393, -11.26763008640078212 ) ) ;
#13811=DIRECTION ( 'NONE',  ( 0.9173788132826626862, 0.000000000000000000, -0.3980152169705242216 ) ) ;
#13828=CIRCLE ( 'NONE', #397, 1.191259999999999097 ) ;
#13829=AXIS2_PLACEMENT_3D ( 'NONE', #6591, #18413, #5665 ) ;
#13831=EDGE_CURVE ( 'NONE', #21627, #5959, #12040, .T. ) ;
#13836=EDGE_LOOP ( 'NONE', ( #10052, #6069, #14686, #16494 ) ) ;
#13840=CARTESIAN_POINT ( 'NONE',  ( 62.90077106633562209, -14.84248999999999974, 8.141649473166729933 ) ) ;
#13847=DIRECTION ( 'NONE',  ( -0.9964481331860213231, 0.000000000000000000, 0.08420877549337311974 ) ) ;
#13860=DIRECTION ( 'NONE',  ( 0.08420877549337300871, 0.000000000000000000, 0.9964481331860212121 ) ) ;
#13864=EDGE_CURVE ( 'NONE', #15795, #17763, #6122, .T. ) ;
#13876=ADVANCED_FACE ( 'NONE', ( #4580, #13107, #4895 ), #18378, .F. ) ;
#13888=CARTESIAN_POINT ( 'NONE',  ( 30.74535937054756829, -1.983739999999999393, -3.684081112461307317 ) ) ;
#13889=VECTOR ( 'NONE', #13926, 1000.000000000000000 ) ;
#13891=PLANE ( 'NONE',  #13244 ) ;
#13903=LINE ( 'NONE', #20600, #153 ) ;
#13912=CARTESIAN_POINT ( 'NONE',  ( 12.13621795668766445, -1.983739999999999393, 4.225309685850866082 ) ) ;
#13917=( NAMED_UNIT ( * ) SI_UNIT ( $, .STERADIAN. ) SOLID_ANGLE_UNIT ( ) );
#13926=DIRECTION ( 'NONE',  ( 0.000000000000000000, 1.000000000000000000, 0.000000000000000000 ) ) ;
#13931=LINE ( 'NONE', #3847, #1530 ) ;
#13933=LINE ( 'NONE', #85, #14123 ) ;
#13936=VERTEX_POINT ( 'NONE', #18592 ) ;
#13963=ORIENTED_EDGE ( 'NONE', *, *, #18264, .T. ) ;
#13967=ORIENTED_EDGE ( 'NONE', *, *, #4217, .T. ) ;
#13971=LINE ( 'NONE', #6969, #19054 ) ;
#13977=CARTESIAN_POINT ( 'NONE',  ( 55.52866846859686234, -3.968114999999999615, -11.12083858657437752 ) ) ;
#13980=ADVANCED_FACE ( 'NONE', ( #13757 ), #21, .T. ) ;
#13982=LINE ( 'NONE', #5537, #2615 ) ;
#13996=VERTEX_POINT ( 'NONE', #20347 ) ;
#13997=EDGE_CURVE ( 'NONE', #2204, #6731, #12090, .T. ) ;
#14001=DIRECTION ( 'NONE',  ( 0.000000000000000000, 1.000000000000000000, 0.000000000000000000 ) ) ;
#14003=EDGE_LOOP ( 'NONE', ( #4804, #2852, #21128, #6254 ) ) ;
#14014=DIRECTION ( 'NONE',  ( 0.000000000000000000, 1.000000000000000000, 0.000000000000000000 ) ) ;
#14022=CARTESIAN_POINT ( 'NONE',  ( 0.000000000000000000, 0.000000000000000000, 0.000000000000000000 ) ) ;
#14024=EDGE_CURVE ( 'NONE', #10465, #4266, #14905, .T. ) ;
#14029=DIRECTION ( 'NONE',  ( 0.000000000000000000, 1.000000000000000000, 0.000000000000000000 ) ) ;
#14035=LINE ( 'NONE', #737, #4366 ) ;
#14051=ORIENTED_EDGE ( 'NONE', *, *, #17949, .T. ) ;
#14055=DIRECTION ( 'NONE',  ( 0.000000000000000000, 1.000000000000000000, 0.000000000000000000 ) ) ;
#14056=DIRECTION ( 'NONE',  ( 0.000000000000000000, 1.000000000000000000, 0.000000000000000000 ) ) ;
#14070=ORIENTED_EDGE ( 'NONE', *, *, #8842, .F. ) ;
#14079=DIRECTION ( 'NONE',  ( -0.9173788132826627972, 0.000000000000000000, 0.3980152169705239440 ) ) ;
#14085=DIRECTION ( 'NONE',  ( 0.000000000000000000, 1.000000000000000000, 0.000000000000000000 ) ) ;
#14088=LINE ( 'NONE', #14310, #10964 ) ;
#14089=LINE ( 'NONE', #16079, #18084 ) ;
#14092=CIRCLE ( 'NONE', #20760, 9.525000000000002132 ) ;
#14108=ORIENTED_EDGE ( 'NONE', *, *, #12684, .T. ) ;
#14111=PLANE ( 'NONE',  #17039 ) ;
#14114=VECTOR ( 'NONE', #3800, 1000.000000000000000 ) ;
#14117=VERTEX_POINT ( 'NONE', #10862 ) ;
#14123=VECTOR ( 'NONE', #6836, 1000.000000000000000 ) ;
#14127=EDGE_CURVE ( 'NONE', #20855, #337, #1102, .T. ) ;
#14129=FACE_OUTER_BOUND ( 'NONE', #17991, .T. ) ;
#14141=CARTESIAN_POINT ( 'NONE',  ( 3.805353748838121053, 34.52875999999999834, -22.18284873352824960 ) ) ;
#14142=ADVANCED_FACE ( 'NONE', ( #686 ), #19031, .T. ) ;
#14145=VERTEX_POINT ( 'NONE', #12538 ) ;
#14148=FACE_OUTER_BOUND ( 'NONE', #19569, .T. ) ;
#14158=EDGE_LOOP ( 'NONE', ( #12763, #7410 ) ) ;
#14166=EDGE_CURVE ( 'NONE', #15906, #8103, #16304, .T. ) ;
#14168=CARTESIAN_POINT ( 'NONE',  ( 12.57635667311951622, -3.968114999999999615, 1.354834321244424267 ) ) ;
#14172=EDGE_LOOP ( 'NONE', ( #3472, #10139, #4174, #16839 ) ) ;
#14189=CARTESIAN_POINT ( 'NONE',  ( -24.20935654380574320, 39.45064500000000152, -25.29247038871795894 ) ) ;
#14193=DIRECTION ( 'NONE',  ( 0.000000000000000000, 1.000000000000000000, 0.000000000000000000 ) ) ;
#14199=DIRECTION ( 'NONE',  ( 0.000000000000000000, 1.000000000000000000, 0.000000000000000000 ) ) ;
#14206=AXIS2_PLACEMENT_3D ( 'NONE', #15834, #17481, #1988 ) ;
#14207=LINE ( 'NONE', #20922, #12409 ) ;
#14210=CARTESIAN_POINT ( 'NONE',  ( 11.56192577415882816, -3.968114999999999615, 4.677561850332325299 ) ) ;
#14227=AXIS2_PLACEMENT_3D ( 'NONE', #19332, #12278, #12174 ) ;
#14234=CARTESIAN_POINT ( 'NONE',  ( 3.360635606688116894, -14.84248999999999974, -20.45316710734507026 ) ) ;
#14244=CARTESIAN_POINT ( 'NONE',  ( 11.11006317807338561, -14.84248999999999974, 0.5252656612939419212 ) ) ;
#14245=VERTEX_POINT ( 'NONE', #21242 ) ;
#14257=ORIENTED_EDGE ( 'NONE', *, *, #10124, .F. ) ;
#14275=DIRECTION ( 'NONE',  ( 0.9964481331860212121, 0.000000000000000000, -0.08420877549337300871 ) ) ;
#14279=DIRECTION ( 'NONE',  ( 0.000000000000000000, 1.000000000000000000, 0.000000000000000000 ) ) ;
#14285=ORIENTED_EDGE ( 'NONE', *, *, #21010, .T. ) ;
#14286=ORIENTED_EDGE ( 'NONE', *, *, #6404, .F. ) ;
#14288=DIRECTION ( 'NONE',  ( 0.000000000000000000, 1.000000000000000000, 0.000000000000000000 ) ) ;
#14293=CARTESIAN_POINT ( 'NONE',  ( 12.13621795668766445, 36.51313500000000545, 4.225309685850866082 ) ) ;
#14296=CARTESIAN_POINT ( 'NONE',  ( -24.21104940531825633, -6.903720000000000745, -25.29232732678598339 ) ) ;
#14297=EDGE_CURVE ( 'NONE', #16776, #15970, #14526, .T. ) ;
#14304=AXIS2_PLACEMENT_3D ( 'NONE', #11307, #9427, #3023 ) ;
#14310=CARTESIAN_POINT ( 'NONE',  ( -16.73439918454169018, -4.609114529603660415, -25.92417111164088084 ) ) ;
#14314=DIRECTION ( 'NONE',  ( -0.08420877549337300871, 0.000000000000000000, -0.9964481331860212121 ) ) ;
#14317=FACE_OUTER_BOUND ( 'NONE', #21430, .T. ) ;
#14324=EDGE_CURVE ( 'NONE', #14947, #21357, #15145, .T. ) ;
#14334=ORIENTED_EDGE ( 'NONE', *, *, #4617, .T. ) ;
#14349=ORIENTED_EDGE ( 'NONE', *, *, #6253, .F. ) ;
#14350=LINE ( 'NONE', #20730, #128 ) ;
#14352=ORIENTED_EDGE ( 'NONE', *, *, #19357, .T. ) ;
#14361=ORIENTED_EDGE ( 'NONE', *, *, #674, .F. ) ;
#14362=ORIENTED_EDGE ( 'NONE', *, *, #1587, .F. ) ;
#14365=CARTESIAN_POINT ( 'NONE',  ( 22.02657784715807665, 36.51313500000000545, -12.98906981665815330 ) ) ;
#14366=VERTEX_POINT ( 'NONE', #14643 ) ;
#14368=ORIENTED_EDGE ( 'NONE', *, *, #11855, .T. ) ;
#14370=EDGE_LOOP ( 'NONE', ( #4288, #9314, #10923, #19659 ) ) ;
#14371=EDGE_CURVE ( 'NONE', #19273, #5598, #1630, .T. ) ;
#14375=DIRECTION ( 'NONE',  ( -0.9964481331860213231, 0.000000000000000000, 0.08420877549337311974 ) ) ;
#14380=LINE ( 'NONE', #21533, #5394 ) ;
#14387=ORIENTED_EDGE ( 'NONE', *, *, #8171, .T. ) ;
#14389=AXIS2_PLACEMENT_3D ( 'NONE', #4583, #17965, #6232 ) ;
#14402=VECTOR ( 'NONE', #2991, 1000.000000000000000 ) ;
#14404=LINE ( 'NONE', #18242, #135 ) ;
#14405=DIRECTION ( 'NONE',  ( 0.2490110332224848289, 0.000000000000000000, -0.9685006480810792739 ) ) ;
#14408=CYLINDRICAL_SURFACE ( 'NONE', #19527, 0.3962400000000000366 ) ;
#14416=EDGE_CURVE ( 'NONE', #16799, #21613, #8822, .T. ) ;
#14428=VERTEX_POINT ( 'NONE', #13810 ) ;
#14460=EDGE_CURVE ( 'NONE', #19233, #17007, #144, .T. ) ;
#14464=FACE_OUTER_BOUND ( 'NONE', #13708, .T. ) ;
#14465=LINE ( 'NONE', #12363, #4161 ) ;
#14471=ORIENTED_EDGE ( 'NONE', *, *, #3722, .F. ) ;
#14476=VERTEX_POINT ( 'NONE', #16947 ) ;
#14481=FACE_OUTER_BOUND ( 'NONE', #18252, .T. ) ;
#14483=FACE_OUTER_BOUND ( 'NONE', #10983, .T. ) ;
#14484=CARTESIAN_POINT ( 'NONE',  ( 19.99312429566830218, -1.983739999999999393, -11.46559883803463720 ) ) ;
#14491=CARTESIAN_POINT ( 'NONE',  ( 3.360635606688116894, 34.52875999999999834, -20.45316710734507026 ) ) ;
#14492=ORIENTED_EDGE ( 'NONE', *, *, #11413, .F. ) ;
#14515=EDGE_CURVE ( 'NONE', #17451, #8841, #10907, .T. ) ;
#14519=CIRCLE ( 'NONE', #9555, 15.47812499999999680 ) ;
#14526=LINE ( 'NONE', #19588, #17366 ) ;
#14548=FACE_OUTER_BOUND ( 'NONE', #11919, .T. ) ;
#14551=CYLINDRICAL_SURFACE ( 'NONE', #16703, 1.191259999999998209 ) ;
#14552=AXIS2_PLACEMENT_3D ( 'NONE', #9190, #14314, #5879 ) ;
#14561=SHAPE_REPRESENTATION_RELATIONSHIP ( 'NONE' , 'NONE' ,  #17083, #13006 ) ;
#14563=CIRCLE ( 'NONE', #20868, 0.7950200000000000600 ) ;
#14564=DIRECTION ( 'NONE',  ( 0.9636276526537417286, 0.000000000000000000, -0.2672484743474500268 ) ) ;
#14572=EDGE_CURVE ( 'NONE', #17145, #6991, #6993, .T. ) ;
#14589=CARTESIAN_POINT ( 'NONE',  ( 21.25660046192028929, 34.52875999999999834, -13.18703856829094079 ) ) ;
#14598=ORIENTED_EDGE ( 'NONE', *, *, #5156, .T. ) ;
#14608=ORIENTED_EDGE ( 'NONE', *, *, #2912, .T. ) ;
#14619=DIRECTION ( 'NONE',  ( 0.08420877549337300871, 0.000000000000000000, 0.9964481331860212121 ) ) ;
#14631=PLANE ( 'NONE',  #19204 ) ;
#14633=CARTESIAN_POINT ( 'NONE',  ( 12.59675778470975516, -14.84248999999999974, -12.54640024901842033 ) ) ;
#14636=CIRCLE ( 'NONE', #8953, 5.158739999999998105 ) ;
#14640=DIRECTION ( 'NONE',  ( 0.000000000000000000, 1.000000000000000000, 0.000000000000000000 ) ) ;
#14643=CARTESIAN_POINT ( 'NONE',  ( 55.52866846859686234, -1.983739999999999393, -11.12083858657437752 ) ) ;
#14651=ORIENTED_EDGE ( 'NONE', *, *, #6005, .T. ) ;
#14656=AXIS2_PLACEMENT_3D ( 'NONE', #11045, #21200, #1083 ) ;
#14666=CARTESIAN_POINT ( 'NONE',  ( 19.99312429566830218, 36.51313500000000545, -11.46559883803463720 ) ) ;
#14668=LINE ( 'NONE', #19708, #5740 ) ;
#14674=CARTESIAN_POINT ( 'NONE',  ( -47.86049599909252805, -5.714364999999999029, -23.29373766372935961 ) ) ;
#14686=ORIENTED_EDGE ( 'NONE', *, *, #3422, .T. ) ;
#14697=CARTESIAN_POINT ( 'NONE',  ( 17.87574706213523612, -3.968114999999999615, -11.18912023382283571 ) ) ;
#14701=ADVANCED_FACE ( 'NONE', ( #6104 ), #9313, .F. ) ;
#14710=ORIENTED_EDGE ( 'NONE', *, *, #15776, .F. ) ;
#14720=EDGE_CURVE ( 'NONE', #9714, #18111, #12547, .T. ) ;
#14726=DIRECTION ( 'NONE',  ( 0.9636276526537417286, 0.000000000000000000, -0.2672484743474500268 ) ) ;
#14734=CARTESIAN_POINT ( 'NONE',  ( -15.40073180482455939, 37.13938632784453375, -10.30507461914819878 ) ) ;
#14751=ORIENTED_EDGE ( 'NONE', *, *, #11852, .F. ) ;
#14752=DIRECTION ( 'NONE',  ( 0.2490110332224836354, 0.000000000000000000, -0.9685006480810794960 ) ) ;
#14755=CARTESIAN_POINT ( 'NONE',  ( 17.30373842852263877, -3.968114999999999615, -12.15706637069277107 ) ) ;
#14771=EDGE_CURVE ( 'NONE', #7624, #14476, #21136, .T. ) ;
#14780=CARTESIAN_POINT ( 'NONE',  ( -18.18961309330695997, -3.266559801243759331, -25.80119252674831998 ) ) ;
#14786=AXIS2_PLACEMENT_3D ( 'NONE', #5475, #3942, #12130 ) ;
#14793=EDGE_LOOP ( 'NONE', ( #12152, #18875, #4808, #5635 ) ) ;
#14801=CARTESIAN_POINT ( 'NONE',  ( 21.45456921355305724, -14.84248999999999974, -13.95701595352872815 ) ) ;
#14804=VECTOR ( 'NONE', #6242, 1000.000000000000000 ) ;
#14832=ORIENTED_EDGE ( 'NONE', *, *, #496, .T. ) ;
#14836=AXIS2_PLACEMENT_3D ( 'NONE', #4152, #16107, #6129 ) ;
#14837=EDGE_CURVE ( 'NONE', #12265, #5398, #8201, .T. ) ;
#14838=EDGE_CURVE ( 'NONE', #21482, #5560, #18258, .T. ) ;
#14840=CARTESIAN_POINT ( 'NONE',  ( -17.01419847615277092, 34.52875999999999834, -25.90052557009608236 ) ) ;
#14843=CARTESIAN_POINT ( 'NONE',  ( 17.02725982432203367, -1.983739999999999393, -14.27444360421403857 ) ) ;
#14847=ORIENTED_EDGE ( 'NONE', *, *, #17803, .F. ) ;
#14852=ORIENTED_EDGE ( 'NONE', *, *, #1564, .T. ) ;
#14859=LINE ( 'NONE', #9967, #17279 ) ;
#14877=ORIENTED_EDGE ( 'NONE', *, *, #6926, .F. ) ;
#14878=LINE ( 'NONE', #6124, #13519 ) ;
#14880=CARTESIAN_POINT ( 'NONE',  ( 3.360635606688116894, -14.84248999999999974, -20.45316710734507026 ) ) ;
#14881=ORIENTED_EDGE ( 'NONE', *, *, #2574, .F. ) ;
#14883=DIRECTION ( 'NONE',  ( 0.08420877549337300871, 0.000000000000000000, 0.9964481331860212121 ) ) ;
#14887=ORIENTED_EDGE ( 'NONE', *, *, #17879, .T. ) ;
#14889=AXIS2_PLACEMENT_3D ( 'NONE', #14666, #18274, #9758 ) ;
#14905=CIRCLE ( 'NONE', #21581, 11.02160133116777985 ) ;
#14910=DIRECTION ( 'NONE',  ( 0.000000000000000000, 1.000000000000000000, 0.000000000000000000 ) ) ;
#14921=ORIENTED_EDGE ( 'NONE', *, *, #2624, .F. ) ;
#14923=EDGE_CURVE ( 'NONE', #16893, #18301, #14859, .T. ) ;
#14924=CARTESIAN_POINT ( 'NONE',  ( 14.05820270259704152, -3.968114999999999615, -15.03781736451272444 ) ) ;
#14927=AXIS2_PLACEMENT_3D ( 'NONE', #9804, #14931, #18224 ) ;
#14929=CIRCLE ( 'NONE', #3972, 1.785937499999999956 ) ;
#14931=DIRECTION ( 'NONE',  ( 0.000000000000000000, 1.000000000000000000, 0.000000000000000000 ) ) ;
#14933=CARTESIAN_POINT ( 'NONE',  ( 62.90077106633562209, 36.51313500000000545, 8.141649473166729933 ) ) ;
#14936=ORIENTED_EDGE ( 'NONE', *, *, #13178, .F. ) ;
#14941=ORIENTED_EDGE ( 'NONE', *, *, #14720, .T. ) ;
#14947=VERTEX_POINT ( 'NONE', #7872 ) ;
#14955=EDGE_CURVE ( 'NONE', #10206, #7846, #13309, .T. ) ;
#14967=CIRCLE ( 'NONE', #18454, 0.7950200000000000600 ) ;
#14978=VECTOR ( 'NONE', #17985, 1000.000000000000000 ) ;
#14979=DIRECTION ( 'NONE',  ( -0.000000000000000000, -1.000000000000000000, 0.000000000000000000 ) ) ;
#14986=LINE ( 'NONE', #15415, #10002 ) ;
#14999=DIRECTION ( 'NONE',  ( -0.000000000000000000, -1.000000000000000000, 0.000000000000000000 ) ) ;
#15000=DIRECTION ( 'NONE',  ( -0.9685006480810792739, 0.000000000000000000, -0.2490110332224846346 ) ) ;
#15002=DIRECTION ( 'NONE',  ( 0.7334850928793759106, 0.6768732144311037091, -0.06198604769977157647 ) ) ;
#15007=EDGE_LOOP ( 'NONE', ( #12975, #14832, #20467, #7126 ) ) ;
#15010=ORIENTED_EDGE ( 'NONE', *, *, #3587, .T. ) ;
#15011=B_SPLINE_CURVE_WITH_KNOTS ( 'NONE', 3,
 ( #338, #15621, #460, #18681 ),
 .UNSPECIFIED., .F., .F.,
 ( 4, 4 ),
 ( 0.000000000000000000, 1.000000000000000000 ),
 .UNSPECIFIED. ) ;
#15024=CARTESIAN_POINT ( 'NONE',  ( -53.00154558624916490, -14.84248999999999974, -22.85927301266823264 ) ) ;
#15032=EDGE_CURVE ( 'NONE', #19233, #16242, #8522, .T. ) ;
#15040=ORIENTED_EDGE ( 'NONE', *, *, #21825, .F. ) ;
#15046=EDGE_LOOP ( 'NONE', ( #13018, #20918, #16756, #8207, #8013, #17139, #8054, #6889, #9467, #9114, #16236, #14051 ) ) ;
#15051=DIRECTION ( 'NONE',  ( 0.9964481331860213231, 0.000000000000000000, -0.08420877549337293932 ) ) ;
#15052=VERTEX_POINT ( 'NONE', #6978 ) ;
#15080=DIRECTION ( 'NONE',  ( -0.000000000000000000, -1.000000000000000000, 0.000000000000000000 ) ) ;
#15083=VECTOR ( 'NONE', #660, 1000.000000000000114 ) ;
#15086=EDGE_CURVE ( 'NONE', #21482, #7846, #1397, .T. ) ;
#15088=DIRECTION ( 'NONE',  ( 0.9685006480810794960, 0.000000000000000000, 0.2490110332224836354 ) ) ;
#15095=LINE ( 'NONE', #21809, #4687 ) ;
#15099=PLANE ( 'NONE',  #9172 ) ;
#15106=CARTESIAN_POINT ( 'NONE',  ( -15.39353573898878658, -4.587157632697119958, -10.30107656633069979 ) ) ;
#15115=ADVANCED_FACE ( 'NONE', ( #3783 ), #20676, .T. ) ;
#15124=ORIENTED_EDGE ( 'NONE', *, *, #437, .F. ) ;
#15128=ORIENTED_EDGE ( 'NONE', *, *, #17854, .F. ) ;
#15130=AXIS2_PLACEMENT_3D ( 'NONE', #3104, #21673, #13296 ) ;
#15131=ORIENTED_EDGE ( 'NONE', *, *, #2574, .T. ) ;
#15141=VERTEX_POINT ( 'NONE', #7093 ) ;
#15145=LINE ( 'NONE', #13480, #6051 ) ;
#15157=ADVANCED_FACE ( 'NONE', ( #17387, #4653, #11072 ), #18144, .F. ) ;
#15164=VERTEX_POINT ( 'NONE', #6296 ) ;
#15167=CARTESIAN_POINT ( 'NONE',  ( 17.79723720954694954, -3.968114999999999615, -14.07647485258271303 ) ) ;
#15169=LINE ( 'NONE', #1444, #7003 ) ;
#15173=DIRECTION ( 'NONE',  ( -0.9685006480810792739, 0.000000000000000000, -0.2490110332224846346 ) ) ;
#15183=ADVANCED_FACE ( 'NONE', ( #18027 ), #16383, .T. ) ;
#15205=EDGE_CURVE ( 'NONE', #3064, #20432, #997, .T. ) ;
#15213=ADVANCED_FACE ( 'NONE', ( #3530 ), #16705, .F. ) ;
#15219=DIRECTION ( 'NONE',  ( -0.9685006480810792739, 0.000000000000000000, -0.2490110332224846346 ) ) ;
#15220=EDGE_LOOP ( 'NONE', ( #14941, #19477, #9874, #3200 ) ) ;
#15242=FACE_OUTER_BOUND ( 'NONE', #6868, .T. ) ;
#15248=CARTESIAN_POINT ( 'NONE',  ( -13.87568970999206108, 34.52875999999999834, -9.457638332870221376 ) ) ;
#15252=ORIENTED_EDGE ( 'NONE', *, *, #19260, .F. ) ;
#15260=ORIENTED_EDGE ( 'NONE', *, *, #4417, .F. ) ;
#15265=DIRECTION ( 'NONE',  ( 0.000000000000000000, 1.000000000000000000, 0.000000000000000000 ) ) ;
#15266=ORIENTED_EDGE ( 'NONE', *, *, #13217, .F. ) ;
#15290=FACE_OUTER_BOUND ( 'NONE', #9585, .T. ) ;
#15294=EDGE_CURVE ( 'NONE', #10693, #18449, #11832, .T. ) ;
#15307=VECTOR ( 'NONE', #14085, 1000.000000000000000 ) ;
#15326=DIRECTION ( 'NONE',  ( -0.3447671952293630548, 0.000000000000000000, -0.9386882235831439658 ) ) ;
#15327=AXIS2_PLACEMENT_3D ( 'NONE', #8738, #7316, #345 ) ;
#15330=ORIENTED_EDGE ( 'NONE', *, *, #1587, .T. ) ;
#15337=DIRECTION ( 'NONE',  ( 0.000000000000000000, 1.000000000000000000, 0.000000000000000000 ) ) ;
#15338=EDGE_LOOP ( 'NONE', ( #1391, #1637, #19785, #3602, #5918, #11037, #3754, #8023, #13505, #5618, #9861, #586, #11286, #10686, #12260, #3164, #12840, #7655, #13248, #12043, #11417 ) ) ;
#15344=DIRECTION ( 'NONE',  ( -0.000000000000000000, -1.000000000000000000, 0.000000000000000000 ) ) ;
#15350=AXIS2_PLACEMENT_3D ( 'NONE', #6953, #16806, #20873 ) ;
#15351=CARTESIAN_POINT ( 'NONE',  ( -22.90596259062238005, 41.43438499999999891, -9.869321627248080375 ) ) ;
#15360=EDGE_CURVE ( 'NONE', #15052, #11891, #6326, .T. ) ;
#15363=CARTESIAN_POINT ( 'NONE',  ( -15.61825442841647593, 37.36444197669704437, -10.42024638160073735 ) ) ;
#15365=EDGE_CURVE ( 'NONE', #227, #6968, #13316, .T. ) ;
#15371=CARTESIAN_POINT ( 'NONE',  ( 13.28822531734660828, 34.52875999999999834, -15.23578611614444078 ) ) ;
#15379=ORIENTED_EDGE ( 'NONE', *, *, #8817, .T. ) ;
#15406=ORIENTED_EDGE ( 'NONE', *, *, #8171, .F. ) ;
#15415=CARTESIAN_POINT ( 'NONE',  ( 11.82678039945931481, 34.52875999999999834, -12.74436900065013667 ) ) ;
#15422=DIRECTION ( 'NONE',  ( 0.000000000000000000, 1.000000000000000000, 0.000000000000000000 ) ) ;
#15445=AXIS2_PLACEMENT_3D ( 'NONE', #7841, #6186, #14288 ) ;
#15456=CYLINDRICAL_SURFACE ( 'NONE', #4520, 1.191259999999999986 ) ;
#15458=EDGE_CURVE ( 'NONE', #7937, #11569, #8875, .T. ) ;
#15460=VECTOR ( 'NONE', #951, 1000.000000000000000 ) ;
#15467=EDGE_CURVE ( 'NONE', #1525, #14117, #10959, .T. ) ;
#15478=EDGE_LOOP ( 'NONE', ( #14070, #15010, #16135, #15128 ) ) ;
#15487=ORIENTED_EDGE ( 'NONE', *, *, #16700, .T. ) ;
#15498=ORIENTED_EDGE ( 'NONE', *, *, #11833, .T. ) ;
#15501=LINE ( 'NONE', #6744, #57 ) ;
#15507=ORIENTED_EDGE ( 'NONE', *, *, #3869, .T. ) ;
#15517=CARTESIAN_POINT ( 'NONE',  ( -15.27766260488554195, 34.52875999999999834, -26.04727837583638461 ) ) ;
#15537=EDGE_LOOP ( 'NONE', ( #15487, #19515, #12253, #9604, #21404, #6346, #1270, #13604, #4952, #19641, #5175, #14877, #19364, #1928, #17804, #549, #7004, #558, #5131, #14598, #16950, #12871, #19629, #8776, #15714, #21661, #2088, #18020 ) ) ;
#15546=VECTOR ( 'NONE', #21554, 1000.000000000000000 ) ;
#15555=EDGE_LOOP ( 'NONE', ( #16013, #20728, #19622, #5783, #17234, #8284, #9166, #15696, #16110, #18307, #11493, #5706 ) ) ;
#15586=ORIENTED_EDGE ( 'NONE', *, *, #17802, .F. ) ;
#15593=AXIS2_PLACEMENT_3D ( 'NONE', #7551, #20919, #12303 ) ;
#15597=CIRCLE ( 'NONE', #3570, 0.7950200000000003930 ) ;
#15600=DIRECTION ( 'NONE',  ( 0.9964481331860213231, 0.000000000000000000, -0.08420877549337293932 ) ) ;
#15603=DIRECTION ( 'NONE',  ( -0.2672484743474505819, 0.000000000000000000, -0.9636276526537416176 ) ) ;
#15615=CYLINDRICAL_SURFACE ( 'NONE', #20167, 0.7950200000000000600 ) ;
#15620=ORIENTED_EDGE ( 'NONE', *, *, #17775, .T. ) ;
#15621=CARTESIAN_POINT ( 'NONE',  ( -15.60052840353961656, -2.331258458467470263, -10.41609846181393451 ) ) ;
#15630=CIRCLE ( 'NONE', #5728, 0.7950200000000003930 ) ;
#15633=CARTESIAN_POINT ( 'NONE',  ( 46.03750000000000142, 34.52875999999999834, -10.31874999999999964 ) ) ;
#15637=AXIS2_PLACEMENT_3D ( 'NONE', #8470, #5058, #20287 ) ;
#15643=DIRECTION ( 'NONE',  ( 0.000000000000000000, 1.000000000000000000, 0.000000000000000000 ) ) ;
#15657=DIRECTION ( 'NONE',  ( -0.2672484743474491942, 0.000000000000000000, -0.9636276526537419507 ) ) ;
#15667=CARTESIAN_POINT ( 'NONE',  ( -22.47451353405102026, -10.87373999999999974, -25.43908013252627853 ) ) ;
#15679=CARTESIAN_POINT ( 'NONE',  ( -22.90596259062238005, -8.889364999999999739, -9.869321627248080375 ) ) ;
#15685=ORIENTED_EDGE ( 'NONE', *, *, #1657, .T. ) ;
#15691=VECTOR ( 'NONE', #7155, 1000.000000000000000 ) ;
#15692=LINE ( 'NONE', #14141, #13889 ) ;
#15696=ORIENTED_EDGE ( 'NONE', *, *, #13997, .F. ) ;
#15697=DIRECTION ( 'NONE',  ( 0.3447671952293626108, 0.000000000000000000, 0.9386882235831439658 ) ) ;
#15699=DIRECTION ( 'NONE',  ( -0.9685006480810794960, 0.000000000000000000, -0.2490110332224836354 ) ) ;
#15714=ORIENTED_EDGE ( 'NONE', *, *, #12213, .T. ) ;
#15719=FACE_OUTER_BOUND ( 'NONE', #19059, .T. ) ;
#15732=CYLINDRICAL_SURFACE ( 'NONE', #14206, 1.785937500000001510 ) ;
#15735=AXIS2_PLACEMENT_3D ( 'NONE', #12049, #13615, #5183 ) ;
#15749=CARTESIAN_POINT ( 'NONE',  ( 11.82678039945931481, -3.968114999999999615, -12.74436900065013667 ) ) ;
#15764=EDGE_LOOP ( 'NONE', ( #11271, #11814, #16712, #5330 ) ) ;
#15766=VECTOR ( 'NONE', #16100, 1000.000000000000000 ) ;
#15776=EDGE_CURVE ( 'NONE', #11237, #10813, #19649, .T. ) ;
#15780=ORIENTED_EDGE ( 'NONE', *, *, #16728, .T. ) ;
#15793=EDGE_CURVE ( 'NONE', #14145, #12588, #8967, .T. ) ;
#15795=VERTEX_POINT ( 'NONE', #16469 ) ;
#15800=ORIENTED_EDGE ( 'NONE', *, *, #1837, .F. ) ;
#15802=DIRECTION ( 'NONE',  ( 0.000000000000000000, 1.000000000000000000, 0.000000000000000000 ) ) ;
#15805=CARTESIAN_POINT ( 'NONE',  ( -47.86112874365709047, -10.87373999999999974, -23.29368419115692035 ) ) ;
#15806=ORIENTED_EDGE ( 'NONE', *, *, #8812, .F. ) ;
#15809=CARTESIAN_POINT ( 'NONE',  ( -46.55773479047372376, -5.714999999999999858, -7.870535429687039120 ) ) ;
#15818=EDGE_LOOP ( 'NONE', ( #2194, #11111, #846, #7677 ) ) ;
#15819=FACE_OUTER_BOUND ( 'NONE', #19757, .T. ) ;
#15827=DIRECTION ( 'NONE',  ( -0.000000000000000000, -1.000000000000000000, 0.000000000000000000 ) ) ;
#15828=CARTESIAN_POINT ( 'NONE',  ( 9.335363283976800375, 36.51313500000000545, -14.20581391854862474 ) ) ;
#15834=CARTESIAN_POINT ( 'NONE',  ( 29.01020070778135818, -14.84248999999999974, -13.85841188422236492 ) ) ;
#15846=DIRECTION ( 'NONE',  ( 0.000000000000000000, 1.000000000000000000, 0.000000000000000000 ) ) ;
#15869=FACE_OUTER_BOUND ( 'NONE', #16289, .T. ) ;
#15870=EDGE_CURVE ( 'NONE', #19449, #10001, #12708, .T. ) ;
#15873=ORIENTED_EDGE ( 'NONE', *, *, #11200, .F. ) ;
#15888=ADVANCED_FACE ( 'NONE', ( #14483 ), #16253, .F. ) ;
#15903=EDGE_CURVE ( 'NONE', #12014, #2636, #13581, .T. ) ;
#15906=VERTEX_POINT ( 'NONE', #6059 ) ;
#15916=CARTESIAN_POINT ( 'NONE',  ( -21.45091887247874851, -8.248365470396340271, -9.992285829511605044 ) ) ;
#15917=FACE_OUTER_BOUND ( 'NONE', #15478, .T. ) ;
#15918=ORIENTED_EDGE ( 'NONE', *, *, #15776, .T. ) ;
#15923=CARTESIAN_POINT ( 'NONE',  ( 13.28822531734660828, -3.968114999999999615, -15.23578611614444078 ) ) ;
#15926=ORIENTED_EDGE ( 'NONE', *, *, #20509, .T. ) ;
#15928=ORIENTED_EDGE ( 'NONE', *, *, #1905, .T. ) ;
#15930=AXIS2_PLACEMENT_3D ( 'NONE', #20793, #9186, #8859 ) ;
#15943=EDGE_CURVE ( 'NONE', #8700, #6063, #14350, .T. ) ;
#15966=CARTESIAN_POINT ( 'NONE',  ( 12.38912331111999343, -14.84248999999999974, 5.137219823516766759 ) ) ;
#15969=VECTOR ( 'NONE', #14055, 1000.000000000000000 ) ;
#15970=VERTEX_POINT ( 'NONE', #2614 ) ;
#15993=CIRCLE ( 'NONE', #18776, 11.02160133116777985 ) ;
#16002=CARTESIAN_POINT ( 'NONE',  ( 55.52866846859686234, 36.51313500000000545, -11.12083858657437752 ) ) ;
#16013=ORIENTED_EDGE ( 'NONE', *, *, #16838, .F. ) ;
#16020=CIRCLE ( 'NONE', #4005, 20.83593750000000000 ) ;
#16023=EDGE_CURVE ( 'NONE', #171, #7176, #5586, .T. ) ;
#16026=EDGE_CURVE ( 'NONE', #10001, #16893, #19070, .T. ) ;
#16027=DIRECTION ( 'NONE',  ( -0.000000000000000000, -1.000000000000000000, 0.000000000000000000 ) ) ;
#16044=CARTESIAN_POINT ( 'NONE',  ( -13.87568970999206108, -1.983739999999999393, -9.457638332870221376 ) ) ;
#16052=EDGE_LOOP ( 'NONE', ( #7411, #6040 ) ) ;
#16055=LINE ( 'NONE', #21214, #9233 ) ;
#16072=DIRECTION ( 'NONE',  ( -0.2490110332224846346, 0.000000000000000000, 0.9685006480810792739 ) ) ;
#16079=CARTESIAN_POINT ( 'NONE',  ( 44.28293121686854761, -3.968114999999999615, -31.08068102505560759 ) ) ;
#16084=ORIENTED_EDGE ( 'NONE', *, *, #21754, .F. ) ;
#16100=DIRECTION ( 'NONE',  ( -0.000000000000000000, -1.000000000000000000, 0.000000000000000000 ) ) ;
#16107=DIRECTION ( 'NONE',  ( 0.000000000000000000, 1.000000000000000000, 0.000000000000000000 ) ) ;
#16110=ORIENTED_EDGE ( 'NONE', *, *, #10973, .T. ) ;
#16116=EDGE_CURVE ( 'NONE', #4266, #20489, #4713, .T. ) ;
#16122=CARTESIAN_POINT ( 'NONE',  ( -15.27935546639805331, 36.51313500000000545, -26.04713531390440906 ) ) ;
#16123=ORIENTED_EDGE ( 'NONE', *, *, #8150, .F. ) ;
#16129=CARTESIAN_POINT ( 'NONE',  ( -15.39353573898878658, 37.13217763270220217, -10.30107656633069979 ) ) ;
#16135=ORIENTED_EDGE ( 'NONE', *, *, #5765, .T. ) ;
#16142=CYLINDRICAL_SURFACE ( 'NONE', #14927, 1.191259999999999319 ) ;
#16147=EDGE_LOOP ( 'NONE', ( #7528, #9573, #21316, #2183 ) ) ;
#16158=CARTESIAN_POINT ( 'NONE',  ( 1.581041518826207248, 36.51313500000000545, -20.30277549736237575 ) ) ;
#16174=DIRECTION ( 'NONE',  ( 0.08420877549337302259, 0.000000000000000000, 0.9964481331860212121 ) ) ;
#16175=CARTESIAN_POINT ( 'NONE',  ( 12.57635667311951622, -1.983739999999999393, 1.354834321244424267 ) ) ;
#16186=VERTEX_POINT ( 'NONE', #13550 ) ;
#16187=EDGE_CURVE ( 'NONE', #9371, #13996, #18515, .T. ) ;
#16192=AXIS2_PLACEMENT_3D ( 'NONE', #19088, #5725, #11136 ) ;
#16194=DIRECTION ( 'NONE',  ( 0.08420877549337302259, 0.000000000000000000, 0.9964481331860212121 ) ) ;
#16207=CARTESIAN_POINT ( 'NONE',  ( -16.14706788831979978, -3.968114999999999615, -25.97380585690919830 ) ) ;
#16222=DIRECTION ( 'NONE',  ( 0.2672484743474500268, 0.000000000000000000, 0.9636276526537417286 ) ) ;
#16227=ORIENTED_EDGE ( 'NONE', *, *, #19747, .T. ) ;
#16231=AXIS2_PLACEMENT_3D ( 'NONE', #12027, #5266, #13811 ) ;
#16232=EDGE_LOOP ( 'NONE', ( #13381, #11022, #13489, #11455 ) ) ;
#16236=ORIENTED_EDGE ( 'NONE', *, *, #1460, .T. ) ;
#16237=ADVANCED_FACE ( 'NONE', ( #7241 ), #2252, .F. ) ;
#16242=VERTEX_POINT ( 'NONE', #17621 ) ;
#16249=AXIS2_PLACEMENT_3D ( 'NONE', #6341, #14999, #18792 ) ;
#16252=DIRECTION ( 'NONE',  ( 0.08420877549337300871, 0.000000000000000000, 0.9964481331860212121 ) ) ;
#16253=CYLINDRICAL_SURFACE ( 'NONE', #1213, 9.524999999999996803 ) ;
#16261=DIRECTION ( 'NONE',  ( -0.000000000000000000, -1.000000000000000000, 0.000000000000000000 ) ) ;
#16268=PLANE ( 'NONE',  #15445 ) ;
#16278=LINE ( 'NONE', #11499, #9672 ) ;
#16289=EDGE_LOOP ( 'NONE', ( #6266, #4199, #8692, #8576 ) ) ;
#16302=ADVANCED_FACE ( 'NONE', ( #5450 ), #13891, .T. ) ;
#16304=CIRCLE ( 'NONE', #14552, 3.175000000000000711 ) ;
#16309=EDGE_CURVE ( 'NONE', #19273, #9683, #3352, .T. ) ;
#16313=CARTESIAN_POINT ( 'NONE',  ( -19.99570496368815142, 42.13594019876639862, -10.11526441440630286 ) ) ;
#16317=CARTESIAN_POINT ( 'NONE',  ( 30.74535937054756829, -95.96551800000000298, -3.684081112461307317 ) ) ;
#16318=CARTESIAN_POINT ( 'NONE',  ( 12.13621795668766445, 34.52875999999999834, 4.225309685850866082 ) ) ;
#16319=ORIENTED_EDGE ( 'NONE', *, *, #3132, .F. ) ;
#16333=ORIENTED_EDGE ( 'NONE', *, *, #15870, .T. ) ;
#16338=AXIS2_PLACEMENT_3D ( 'NONE', #520, #10697, #4167 ) ;
#16351=VERTEX_POINT ( 'NONE', #2474 ) ;
#16354=ORIENTED_EDGE ( 'NONE', *, *, #18578, .T. ) ;
#16360=DIRECTION ( 'NONE',  ( -0.9964481331860213231, 0.000000000000000000, 0.08420877549337293932 ) ) ;
#16363=ORIENTED_EDGE ( 'NONE', *, *, #16309, .F. ) ;
#16371=ORIENTED_EDGE ( 'NONE', *, *, #16728, .F. ) ;
#16379=CIRCLE ( 'NONE', #4376, 9.524999999999996803 ) ;
#16383=CYLINDRICAL_SURFACE ( 'NONE', #10929, 5.158739999999998105 ) ;
#16386=CARTESIAN_POINT ( 'NONE',  ( 9.828862065001116477, 36.51313500000000545, -16.12522240043857025 ) ) ;
#16389=CARTESIAN_POINT ( 'NONE',  ( 9.907371917564091746, 36.51313500000000545, -13.23786778167655243 ) ) ;
#16397=VERTEX_POINT ( 'NONE', #13207 ) ;
#16401=ORIENTED_EDGE ( 'NONE', *, *, #21481, .T. ) ;
#16403=DIRECTION ( 'NONE',  ( -0.000000000000000000, -1.000000000000000000, 0.000000000000000000 ) ) ;
#16412=EDGE_CURVE ( 'NONE', #7070, #21386, #1911, .T. ) ;
#16418=CARTESIAN_POINT ( 'NONE',  ( -22.75431282566211522, -8.248365470396340271, -25.41543459098148716 ) ) ;
#16424=DIRECTION ( 'NONE',  ( 0.000000000000000000, 1.000000000000000000, 0.000000000000000000 ) ) ;
#16435=ORIENTED_EDGE ( 'NONE', *, *, #6271, .F. ) ;
#16446=EDGE_CURVE ( 'NONE', #12265, #5334, #17951, .T. ) ;
#16449=VECTOR ( 'NONE', #16882, 1000.000000000000000 ) ;
#16451=CARTESIAN_POINT ( 'NONE',  ( 3.360635606688116894, -1.983739999999999393, -20.45316710734507026 ) ) ;
#16469=CARTESIAN_POINT ( 'NONE',  ( -24.20935654380574320, -8.889364999999999739, -25.29247038871795894 ) ) ;
#16474=DIRECTION ( 'NONE',  ( -0.2490110332224857170, 0.000000000000000000, 0.9685006480810790519 ) ) ;
#16483=ORIENTED_EDGE ( 'NONE', *, *, #15458, .F. ) ;
#16484=EDGE_CURVE ( 'NONE', #2732, #6731, #21695, .T. ) ;
#16493=VECTOR ( 'NONE', #12613, 1000.000000000000000 ) ;
#16494=ORIENTED_EDGE ( 'NONE', *, *, #21481, .F. ) ;
#16500=DIRECTION ( 'NONE',  ( 0.000000000000000000, 1.000000000000000000, 0.000000000000000000 ) ) ;
#16503=EDGE_LOOP ( 'NONE', ( #7138, #3886, #15379, #14108 ) ) ;
#16511=CARTESIAN_POINT ( 'NONE',  ( 11.82678039945931481, 36.51313500000000545, -12.74436900065013667 ) ) ;
#16518=CARTESIAN_POINT ( 'NONE',  ( -24.20935654380574320, -8.889364999999999739, -25.29247038871795894 ) ) ;
#16521=DIRECTION ( 'NONE',  ( 0.000000000000000000, 1.000000000000000000, 0.000000000000000000 ) ) ;
#16522=ADVANCED_FACE ( 'NONE', ( #11198 ), #2586, .T. ) ;
#16525=FACE_OUTER_BOUND ( 'NONE', #21309, .T. ) ;
#16528=ORIENTED_EDGE ( 'NONE', *, *, #18379, .T. ) ;
#16533=EDGE_CURVE ( 'NONE', #1298, #9903, #11520, .T. ) ;
#16552=ORIENTED_EDGE ( 'NONE', *, *, #3097, .F. ) ;
#16555=DIRECTION ( 'NONE',  ( -0.9685006480810792739, 0.000000000000000000, -0.2490110332224846346 ) ) ;
#16587=LINE ( 'NONE', #19883, #14402 ) ;
#16595=CARTESIAN_POINT ( 'NONE',  ( 17.02725982432203367, -3.968114999999999615, -14.27444360421403857 ) ) ;
#16606=CARTESIAN_POINT ( 'NONE',  ( -15.27766260488554195, -1.983739999999999393, -26.04727837583638461 ) ) ;
#16622=EDGE_CURVE ( 'NONE', #13681, #21107, #6977, .T. ) ;
#16626=FACE_OUTER_BOUND ( 'NONE', #11882, .T. ) ;
#16627=DIRECTION ( 'NONE',  ( 0.000000000000000000, 1.000000000000000000, 0.000000000000000000 ) ) ;
#16631=VECTOR ( 'NONE', #19419, 1000.000000000000114 ) ;
#16638=ORIENTED_EDGE ( 'NONE', *, *, #21103, .T. ) ;
#16647=VECTOR ( 'NONE', #2713, 1000.000000000000000 ) ;
#16659=CARTESIAN_POINT ( 'NONE',  ( 36.54633153140314761, -1.983739999999999393, -9.516661413425623550 ) ) ;
#16666=ORIENTED_EDGE ( 'NONE', *, *, #18950, .T. ) ;
#16669=VECTOR ( 'NONE', #15827, 1000.000000000000000 ) ;
#16685=CIRCLE ( 'NONE', #16704, 15.47812499999999680 ) ;
#16688=DIRECTION ( 'NONE',  ( -0.9685006480810792739, 0.000000000000000000, -0.2490110332224846346 ) ) ;
#16695=VERTEX_POINT ( 'NONE', #16927 ) ;
#16700=EDGE_CURVE ( 'NONE', #17229, #6182, #16731, .T. ) ;
#16703=AXIS2_PLACEMENT_3D ( 'NONE', #16317, #7894, #18074 ) ;
#16704=AXIS2_PLACEMENT_3D ( 'NONE', #12838, #13054, #21098 ) ;
#16705=PLANE ( 'NONE',  #11298 ) ;
#16707=CARTESIAN_POINT ( 'NONE',  ( -22.90596259062238005, -8.889364999999999739, -9.869321627248080375 ) ) ;
#16712=ORIENTED_EDGE ( 'NONE', *, *, #1979, .F. ) ;
#16714=CARTESIAN_POINT ( 'NONE',  ( 13.28822531734660828, 36.51313500000000545, -15.23578611614444078 ) ) ;
#16727=AXIS2_PLACEMENT_3D ( 'NONE', #17329, #8694, #15697 ) ;
#16728=EDGE_CURVE ( 'NONE', #20833, #17882, #4794, .T. ) ;
#16731=CIRCLE ( 'NONE', #6483, 3.970019999999997662 ) ;
#16734=CARTESIAN_POINT ( 'NONE',  ( -15.41509608936259035, -4.609114529603660415, -10.31276839742836415 ) ) ;
#16741=CIRCLE ( 'NONE', #4734, 9.525000000000002132 ) ;
#16745=DIRECTION ( 'NONE',  ( -0.000000000000000000, -1.000000000000000000, 0.000000000000000000 ) ) ;
#16751=FACE_OUTER_BOUND ( 'NONE', #7302, .T. ) ;
#16756=ORIENTED_EDGE ( 'NONE', *, *, #20360, .T. ) ;
#16758=AXIS2_PLACEMENT_3D ( 'NONE', #383, #10336, #8668 ) ;
#16764=AXIS2_PLACEMENT_3D ( 'NONE', #7771, #18170, #6321 ) ;
#16772=ORIENTED_EDGE ( 'NONE', *, *, #3867, .T. ) ;
#16776=VERTEX_POINT ( 'NONE', #13634 ) ;
#16778=ORIENTED_EDGE ( 'NONE', *, *, #18379, .F. ) ;
#16782=ORIENTED_EDGE ( 'NONE', *, *, #339, .T. ) ;
#16792=EDGE_CURVE ( 'NONE', #2731, #6613, #2957, .T. ) ;
#16793=LINE ( 'NONE', #13376, #19719 ) ;
#16795=ORIENTED_EDGE ( 'NONE', *, *, #20748, .F. ) ;
#16799=VERTEX_POINT ( 'NONE', #19140 ) ;
#16801=ADVANCED_FACE ( 'NONE', ( #10634 ), #8965, .T. ) ;
#16802=ORIENTED_EDGE ( 'NONE', *, *, #14515, .T. ) ;
#16806=DIRECTION ( 'NONE',  ( -0.000000000000000000, -1.000000000000000000, 0.000000000000000000 ) ) ;
#16816=DIRECTION ( 'NONE',  ( 0.000000000000000000, 1.000000000000000000, 0.000000000000000000 ) ) ;
#16824=ADVANCED_FACE ( 'NONE', ( #1997 ), #12524, .T. ) ;
#16827=AXIS2_PLACEMENT_3D ( 'NONE', #6126, #17861, #19824 ) ;
#16836=EDGE_CURVE ( 'NONE', #2732, #8399, #6113, .T. ) ;
#16838=EDGE_CURVE ( 'NONE', #5344, #20691, #3893, .T. ) ;
#16839=ORIENTED_EDGE ( 'NONE', *, *, #15086, .F. ) ;
#16842=DIRECTION ( 'NONE',  ( 0.2490110332224857170, 0.000000000000000000, -0.9685006480810790519 ) ) ;
#16849=FACE_OUTER_BOUND ( 'NONE', #17840, .T. ) ;
#16850=VERTEX_POINT ( 'NONE', #13977 ) ;
#16870=DIRECTION ( 'NONE',  ( 0.7334850928793775759, 0.6768732144311021548, -0.06198604769976992501 ) ) ;
#16878=CARTESIAN_POINT ( 'NONE',  ( -22.75431282566211522, 40.79338547039380103, -25.41543459098148716 ) ) ;
#16882=DIRECTION ( 'NONE',  ( -0.000000000000000000, -1.000000000000000000, 0.000000000000000000 ) ) ;
#16884=EDGE_CURVE ( 'NONE', #7791, #14366, #16379, .T. ) ;
#16887=LINE ( 'NONE', #20850, #12091 ) ;
#16893=VERTEX_POINT ( 'NONE', #12293 ) ;
#16912=LINE ( 'NONE', #20104, #20876 ) ;
#16915=ORIENTED_EDGE ( 'NONE', *, *, #1924, .T. ) ;
#16927=CARTESIAN_POINT ( 'NONE',  ( 17.87574706213523612, 36.51313500000000545, -11.18912023382283571 ) ) ;
#16931=CARTESIAN_POINT ( 'NONE',  ( 12.02474915109715603, 36.51313500000000545, -13.51434638588835391 ) ) ;
#16936=DIRECTION ( 'NONE',  ( 0.000000000000000000, 1.000000000000000000, 0.000000000000000000 ) ) ;
#16940=EDGE_LOOP ( 'NONE', ( #7625, #18525, #11348, #7911 ) ) ;
#16947=CARTESIAN_POINT ( 'NONE',  ( 28.56548256563643662, -1.983739999999999393, -12.12873025803960658 ) ) ;
#16950=ORIENTED_EDGE ( 'NONE', *, *, #21445, .T. ) ;
#16956=EDGE_CURVE ( 'NONE', #374, #8103, #8361, .T. ) ;
#16976=CARTESIAN_POINT ( 'NONE',  ( 17.22522857595987844, 36.51313500000000545, -15.04442098945225403 ) ) ;
#16979=VECTOR ( 'NONE', #369, 1000.000000000000000 ) ;
#16985=EDGE_CURVE ( 'NONE', #12465, #2216, #17070, .T. ) ;
#16997=DIRECTION ( 'NONE',  ( 0.000000000000000000, 1.000000000000000000, 0.000000000000000000 ) ) ;
#16999=DIRECTION ( 'NONE',  ( 0.000000000000000000, 1.000000000000000000, 0.000000000000000000 ) ) ;
#17007=VERTEX_POINT ( 'NONE', #19348 ) ;
#17009=FACE_OUTER_BOUND ( 'NONE', #18831, .T. ) ;
#17013=CIRCLE ( 'NONE', #5717, 9.524999999999996803 ) ;
#17020=CARTESIAN_POINT ( 'NONE',  ( 13.28822531734660828, 36.51313500000000545, -15.23578611614444078 ) ) ;
#17023=ORIENTED_EDGE ( 'NONE', *, *, #2288, .F. ) ;
#17025=DIRECTION ( 'NONE',  ( 0.000000000000000000, 1.000000000000000000, 0.000000000000000000 ) ) ;
#17034=ORIENTED_EDGE ( 'NONE', *, *, #13831, .F. ) ;
#17039=AXIS2_PLACEMENT_3D ( 'NONE', #15667, #20816, #20943 ) ;
#17052=DIRECTION ( 'NONE',  ( 0.000000000000000000, 1.000000000000000000, 0.000000000000000000 ) ) ;
#17057=EDGE_CURVE ( 'NONE', #10171, #13681, #12625, .T. ) ;
#17070=CIRCLE ( 'NONE', #20955, 0.7950200000000000600 ) ;
#17083=SHAPE_REPRESENTATION ( 'Ratchet Operating Handle', ( #2234 ), #3303 ) ;
#17086=VECTOR ( 'NONE', #728, 1000.000000000000000 ) ;
#17088=ORIENTED_EDGE ( 'NONE', *, *, #17057, .T. ) ;
#17090=CARTESIAN_POINT ( 'NONE',  ( 18.07371581377308800, -95.96551800000000298, -11.95909761906105473 ) ) ;
#17092=LINE ( 'NONE', #16976, #1434 ) ;
#17097=ORIENTED_EDGE ( 'NONE', *, *, #9250, .F. ) ;
#17101=CYLINDRICAL_SURFACE ( 'NONE', #11786, 0.7950200000000000600 ) ;
#17102=ORIENTED_EDGE ( 'NONE', *, *, #5715, .F. ) ;
#17125=DIRECTION ( 'NONE',  ( 0.000000000000000000, 1.000000000000000000, 0.000000000000000000 ) ) ;
#17129=DIRECTION ( 'NONE',  ( -0.9964481331860212121, 0.000000000000000000, 0.08420877549337305035 ) ) ;
#17136=DIRECTION ( 'NONE',  ( 0.2490110332224848289, 0.000000000000000000, -0.9685006480810792739 ) ) ;
#17139=ORIENTED_EDGE ( 'NONE', *, *, #12051, .T. ) ;
#17145=VERTEX_POINT ( 'NONE', #403 ) ;
#17146=EDGE_CURVE ( 'NONE', #16397, #19794, #10358, .T. ) ;
#17150=ORIENTED_EDGE ( 'NONE', *, *, #4298, .F. ) ;
#17164=DIRECTION ( 'NONE',  ( -0.9173788132826627972, 0.000000000000000000, 0.3980152169705239440 ) ) ;
#17187=CARTESIAN_POINT ( 'NONE',  ( 30.42699695299585017, 36.51313500000000545, -4.832012189960551041 ) ) ;
#17188=ADVANCED_FACE ( 'NONE', ( #15242 ), #17101, .F. ) ;
#17198=ORIENTED_EDGE ( 'NONE', *, *, #4494, .T. ) ;
#17200=FACE_OUTER_BOUND ( 'NONE', #11442, .T. ) ;
#17203=CARTESIAN_POINT ( 'NONE',  ( 12.02474915109715603, -95.96551800000000298, -13.51434638588835391 ) ) ;
#17208=FACE_OUTER_BOUND ( 'NONE', #5395, .T. ) ;
#17214=EDGE_CURVE ( 'NONE', #21739, #7796, #14636, .T. ) ;
#17221=EDGE_LOOP ( 'NONE', ( #19612, #6541, #17740, #12137 ) ) ;
#17229=VERTEX_POINT ( 'NONE', #11905 ) ;
#17234=ORIENTED_EDGE ( 'NONE', *, *, #11200, .T. ) ;
#17236=EDGE_CURVE ( 'NONE', #16695, #19840, #10013, .T. ) ;
#17239=CARTESIAN_POINT ( 'NONE',  ( -22.90596259062238005, -6.905625000000000568, -9.869321627248080375 ) ) ;
#17240=DIRECTION ( 'NONE',  ( -0.3447671952293630548, 0.000000000000000000, -0.9386882235831439658 ) ) ;
#17245=ORIENTED_EDGE ( 'NONE', *, *, #14166, .F. ) ;
#17252=CYLINDRICAL_SURFACE ( 'NONE', #12068, 1.785937499999999512 ) ;
#17257=VECTOR ( 'NONE', #6863, 1000.000000000000114 ) ;
#17260=DIRECTION ( 'NONE',  ( 0.7334850928793773539, -0.6768732144311023768, -0.06198604769976947398 ) ) ;
#17263=DIRECTION ( 'NONE',  ( 0.000000000000000000, 1.000000000000000000, 0.000000000000000000 ) ) ;
#17264=EDGE_CURVE ( 'NONE', #3845, #18633, #20501, .T. ) ;
#17272=DIRECTION ( 'NONE',  ( 0.08420877549337300871, 0.000000000000000000, 0.9964481331860212121 ) ) ;
#17279=VECTOR ( 'NONE', #3345, 1000.000000000000114 ) ;
#17284=CARTESIAN_POINT ( 'NONE',  ( 9.137394532338957376, -14.84248999999999974, -13.43583653331040750 ) ) ;
#17302=FACE_OUTER_BOUND ( 'NONE', #1862, .T. ) ;
#17313=CARTESIAN_POINT ( 'NONE',  ( -17.01419847615277092, -1.983739999999999393, -25.90052557009608236 ) ) ;
#17320=DIRECTION ( 'NONE',  ( 0.2490110332224848289, 0.000000000000000000, -0.9685006480810792739 ) ) ;
#17325=AXIS2_PLACEMENT_3D ( 'NONE', #4803, #19606, #16424 ) ;
#17329=CARTESIAN_POINT ( 'NONE',  ( 55.81697695389291169, 34.52875999999999834, -11.14520323105768362 ) ) ;
#17330=CARTESIAN_POINT ( 'NONE',  ( -14.39647200192766441, 34.52875999999985623, -9.747027169376242028 ) ) ;
#17340=DIRECTION ( 'NONE',  ( -0.9964481331860212121, 0.000000000000000000, 0.08420877549337300871 ) ) ;
#17358=CARTESIAN_POINT ( 'NONE',  ( 20.76310168089343478, -3.968114999999999615, -11.26763008640078212 ) ) ;
#17362=VERTEX_POINT ( 'NONE', #8028 ) ;
#17366=VECTOR ( 'NONE', #3013, 1000.000000000000000 ) ;
#17387=FACE_BOUND ( 'NONE', #6633, .T. ) ;
#17403=EDGE_CURVE ( 'NONE', #5334, #2409, #10165, .T. ) ;
#17411=DIRECTION ( 'NONE',  ( -0.9964481331860212121, 0.000000000000000000, 0.08420877549337302259 ) ) ;
#17414=AXIS2_PLACEMENT_3D ( 'NONE', #7777, #3030, #2700 ) ;
#17428=CARTESIAN_POINT ( 'NONE',  ( 46.03750000000000142, 36.51313500000000545, -10.31874999999999964 ) ) ;
#17439=CIRCLE ( 'NONE', #13206, 1.785937499999998179 ) ;
#17447=CARTESIAN_POINT ( 'NONE',  ( 55.52866846859685523, -14.84248999999999974, -11.12083858657437752 ) ) ;
#17448=DIRECTION ( 'NONE',  ( 0.000000000000000000, 1.000000000000000000, 0.000000000000000000 ) ) ;
#17450=ORIENTED_EDGE ( 'NONE', *, *, #8716, .T. ) ;
#17451=VERTEX_POINT ( 'NONE', #14589 ) ;
#17454=CARTESIAN_POINT ( 'NONE',  ( 17.30373842852263877, -3.968114999999999615, -12.15706637069277107 ) ) ;
#17458=ORIENTED_EDGE ( 'NONE', *, *, #6125, .F. ) ;
#17466=LINE ( 'NONE', #17358, #20624 ) ;
#17468=VERTEX_POINT ( 'NONE', #8454 ) ;
#17476=ORIENTED_EDGE ( 'NONE', *, *, #6005, .F. ) ;
#17481=DIRECTION ( 'NONE',  ( 0.000000000000000000, 1.000000000000000000, 0.000000000000000000 ) ) ;
#17483=ORIENTED_EDGE ( 'NONE', *, *, #4121, .T. ) ;
#17484=AXIS2_PLACEMENT_3D ( 'NONE', #9046, #14279, #9152 ) ;
#17485=ORIENTED_EDGE ( 'NONE', *, *, #14460, .T. ) ;
#17505=EDGE_CURVE ( 'NONE', #4458, #15970, #9891, .T. ) ;
#17509=FACE_OUTER_BOUND ( 'NONE', #1318, .T. ) ;
#17513=ORIENTED_EDGE ( 'NONE', *, *, #1932, .F. ) ;
#17514=AXIS2_PLACEMENT_3D ( 'NONE', #5116, #355, #17052 ) ;
#17516=DIRECTION ( 'NONE',  ( 0.000000000000000000, 1.000000000000000000, 0.000000000000000000 ) ) ;
#17520=ADVANCED_FACE ( 'NONE', ( #4729 ), #13458, .T. ) ;
#17532=CARTESIAN_POINT ( 'NONE',  ( 12.13621795668766445, -3.968114999999999615, 4.225309685850866082 ) ) ;
#17533=ORIENTED_EDGE ( 'NONE', *, *, #15793, .T. ) ;
#17535=DIRECTION ( 'NONE',  ( 0.000000000000000000, 1.000000000000000000, 0.000000000000000000 ) ) ;
#17538=CARTESIAN_POINT ( 'NONE',  ( 14.05820270259704152, 128.5105379999999968, -15.03781736451272444 ) ) ;
#17552=AXIS2_PLACEMENT_3D ( 'NONE', #21763, #14726, #11492 ) ;
#17553=DIRECTION ( 'NONE',  ( 0.000000000000000000, 1.000000000000000000, 0.000000000000000000 ) ) ;
#17554=CYLINDRICAL_SURFACE ( 'NONE', #9782, 11.02160133116777452 ) ;
#17556=LINE ( 'NONE', #5722, #12496 ) ;
#17560=VERTEX_POINT ( 'NONE', #21630 ) ;
#17562=LINE ( 'NONE', #19315, #382 ) ;
#17563=ORIENTED_EDGE ( 'NONE', *, *, #21197, .T. ) ;
#17570=ADVANCED_FACE ( 'NONE', ( #18418 ), #19855, .T. ) ;
#17577=DIRECTION ( 'NONE',  ( 0.000000000000000000, 1.000000000000000000, 0.000000000000000000 ) ) ;
#17609=VECTOR ( 'NONE', #8548, 1000.000000000000000 ) ;
#17617=EDGE_CURVE ( 'NONE', #11228, #8566, #8437, .T. ) ;
#17621=CARTESIAN_POINT ( 'NONE',  ( 9.828862065001116477, -3.968114999999999615, -16.12522240043857025 ) ) ;
#17638=AXIS2_PLACEMENT_3D ( 'NONE', #14234, #7576, #9219 ) ;
#17639=DIRECTION ( 'NONE',  ( -0.9685006480810792739, 0.000000000000000000, -0.2490110332224846346 ) ) ;
#17644=DIRECTION ( 'NONE',  ( 1.000000000000000000, 0.000000000000000000, 0.000000000000000000 ) ) ;
#17646=DIRECTION ( 'NONE',  ( -0.08420877549337300871, 0.000000000000000000, -0.9964481331860212121 ) ) ;
#17649=VECTOR ( 'NONE', #1478, 1000.000000000000000 ) ;
#17657=CARTESIAN_POINT ( 'NONE',  ( 11.82678039945931481, -3.968114999999999615, -12.74436900065013667 ) ) ;
#17662=VECTOR ( 'NONE', #10116, 1000.000000000000000 ) ;
#17672=ORIENTED_EDGE ( 'NONE', *, *, #15360, .F. ) ;
#17673=EDGE_CURVE ( 'NONE', #20432, #4259, #18036, .T. ) ;
#17680=DIRECTION ( 'NONE',  ( 0.000000000000000000, 1.000000000000000000, 0.000000000000000000 ) ) ;
#17681=DIRECTION ( 'NONE',  ( -0.9685006480810792739, 0.000000000000000000, -0.2490110332224846346 ) ) ;
#17689=LINE ( 'NONE', #17807, #17739 ) ;
#17690=CARTESIAN_POINT ( 'NONE',  ( 56.47666780297049627, 36.51313500000000545, 1.109116340531466127 ) ) ;
#17708=AXIS2_PLACEMENT_3D ( 'NONE', #21385, #21719, #15002 ) ;
#17712=DIRECTION ( 'NONE',  ( -0.000000000000000000, -1.000000000000000000, 0.000000000000000000 ) ) ;
#17713=DIRECTION ( 'NONE',  ( -0.000000000000000000, -1.000000000000000000, 0.000000000000000000 ) ) ;
#17724=AXIS2_PLACEMENT_3D ( 'NONE', #10756, #2349, #2459 ) ;
#17738=AXIS2_PLACEMENT_3D ( 'NONE', #7719, #9480, #1080 ) ;
#17739=VECTOR ( 'NONE', #5847, 1000.000000000000000 ) ;
#17740=ORIENTED_EDGE ( 'NONE', *, *, #12211, .F. ) ;
#17748=EDGE_CURVE ( 'NONE', #8949, #6430, #10212, .T. ) ;
#17752=CYLINDRICAL_SURFACE ( 'NONE', #17638, 1.785937499999999512 ) ;
#17763=VERTEX_POINT ( 'NONE', #7019 ) ;
#17765=AXIS2_PLACEMENT_3D ( 'NONE', #17090, #12230, #2271 ) ;
#17768=AXIS2_PLACEMENT_3D ( 'NONE', #18965, #14029, #17320 ) ;
#17775=EDGE_CURVE ( 'NONE', #5934, #8566, #20377, .T. ) ;
#17785=CARTESIAN_POINT ( 'NONE',  ( -13.87747867115857936, 36.51313500000000545, -9.458632424640695646 ) ) ;
#17788=DIRECTION ( 'NONE',  ( 0.2490110332224857170, 0.000000000000000000, -0.9685006480810790519 ) ) ;
#17797=CIRCLE ( 'NONE', #19550, 0.7950200000000003930 ) ;
#17798=CARTESIAN_POINT ( 'NONE',  ( 9.256853431388732290, 36.51313500000000545, -17.09316853730597074 ) ) ;
#17802=EDGE_CURVE ( 'NONE', #20069, #12648, #18952, .T. ) ;
#17803=EDGE_CURVE ( 'NONE', #19273, #13378, #4586, .T. ) ;
#17804=ORIENTED_EDGE ( 'NONE', *, *, #11225, .T. ) ;
#17807=CARTESIAN_POINT ( 'NONE',  ( 14.25617145423489696, -1.983739999999999393, -15.80779474975094168 ) ) ;
#17818=ORIENTED_EDGE ( 'NONE', *, *, #5715, .T. ) ;
#17833=EDGE_CURVE ( 'NONE', #374, #17763, #6732, .T. ) ;
#17834=DIRECTION ( 'NONE',  ( 0.9636276526537417286, 0.000000000000000000, -0.2672484743474499158 ) ) ;
#17840=EDGE_LOOP ( 'NONE', ( #13063, #20245, #14387, #615 ) ) ;
#17843=VERTEX_POINT ( 'NONE', #12787 ) ;
#17850=AXIS2_PLACEMENT_3D ( 'NONE', #14484, #21530, #11256 ) ;
#17854=EDGE_CURVE ( 'NONE', #21307, #2549, #14519, .T. ) ;
#17855=CARTESIAN_POINT ( 'NONE',  ( 1.581041518826207248, -1.983739999999999393, -20.30277549736237575 ) ) ;
#17860=CARTESIAN_POINT ( 'NONE',  ( -13.87568970999206108, 34.52875999999999834, -9.457638332870221376 ) ) ;
#17861=DIRECTION ( 'NONE',  ( -0.08420877549337300871, 0.000000000000000000, -0.9964481331860212121 ) ) ;
#17868=CYLINDRICAL_SURFACE ( 'NONE', #9922, 0.7950200000000000600 ) ;
#17873=ORIENTED_EDGE ( 'NONE', *, *, #4121, .F. ) ;
#17879=EDGE_CURVE ( 'NONE', #9783, #17843, #13069, .T. ) ;
#17882=VERTEX_POINT ( 'NONE', #19290 ) ;
#17900=CARTESIAN_POINT ( 'NONE',  ( -13.97426865170217702, -5.953760000000000829, -10.62412961436650249 ) ) ;
#17905=DIRECTION ( 'NONE',  ( 0.000000000000000000, 1.000000000000000000, 0.000000000000000000 ) ) ;
#17910=ORIENTED_EDGE ( 'NONE', *, *, #8551, .T. ) ;
#17914=DIRECTION ( 'NONE',  ( 0.000000000000000000, 1.000000000000000000, 0.000000000000000000 ) ) ;
#17921=EDGE_CURVE ( 'NONE', #12395, #21254, #18682, .T. ) ;
#17926=AXIS2_PLACEMENT_3D ( 'NONE', #19535, #9359, #3958 ) ;
#17938=ORIENTED_EDGE ( 'NONE', *, *, #21197, .F. ) ;
#17942=CARTESIAN_POINT ( 'NONE',  ( 12.13621795668766445, -1.983739999999999393, 4.225309685850866082 ) ) ;
#17947=ORIENTED_EDGE ( 'NONE', *, *, #21078, .T. ) ;
#17949=EDGE_CURVE ( 'NONE', #19935, #11383, #7684, .T. ) ;
#17951=LINE ( 'NONE', #1246, #19214 ) ;
#17960=PLANE ( 'NONE',  #422 ) ;
#17965=DIRECTION ( 'NONE',  ( 0.000000000000000000, 1.000000000000000000, 0.000000000000000000 ) ) ;
#17983=CIRCLE ( 'NONE', #20075, 1.785937499999998179 ) ;
#17985=DIRECTION ( 'NONE',  ( 0.000000000000000000, 1.000000000000000000, 0.000000000000000000 ) ) ;
#17987=ORIENTED_EDGE ( 'NONE', *, *, #19137, .T. ) ;
#17991=EDGE_LOOP ( 'NONE', ( #8958, #13273, #14361, #8623 ) ) ;
#17999=CIRCLE ( 'NONE', #2102, 3.174999999999997158 ) ;
#18009=CARTESIAN_POINT ( 'NONE',  ( -16.07247711516169275, 37.85422182005619618, -10.44681224123558039 ) ) ;
#18020=ORIENTED_EDGE ( 'NONE', *, *, #11699, .T. ) ;
#18022=EDGE_CURVE ( 'NONE', #13041, #6616, #8798, .T. ) ;
#18024=EDGE_CURVE ( 'NONE', #18743, #19312, #17999, .T. ) ;
#18027=FACE_OUTER_BOUND ( 'NONE', #9003, .T. ) ;
#18036=CIRCLE ( 'NONE', #1780, 20.83593750000000000 ) ;
#18039=DIRECTION ( 'NONE',  ( 0.000000000000000000, 1.000000000000000000, 0.000000000000000000 ) ) ;
#18041=ADVANCED_FACE ( 'NONE', ( #8004 ), #15099, .T. ) ;
#18059=AXIS2_PLACEMENT_3D ( 'NONE', #5785, #12543, #19268 ) ;
#18061=DIRECTION ( 'NONE',  ( -0.2672484743474500268, 0.000000000000000000, -0.9636276526537417286 ) ) ;
#18074=DIRECTION ( 'NONE',  ( 0.9173788132826626862, 0.000000000000000000, -0.3980152169705242216 ) ) ;
#18078=DIRECTION ( 'NONE',  ( 0.2490110332224848289, 0.000000000000000000, -0.9685006480810792739 ) ) ;
#18084=VECTOR ( 'NONE', #4453, 1000.000000000000000 ) ;
#18085=VECTOR ( 'NONE', #17125, 1000.000000000000000 ) ;
#18089=VECTOR ( 'NONE', #3739, 1000.000000000000114 ) ;
#18090=ORIENTED_EDGE ( 'NONE', *, *, #2912, .F. ) ;
#18095=AXIS2_PLACEMENT_3D ( 'NONE', #6714, #13470, #5255 ) ;
#18100=LINE ( 'NONE', #2959, #14978 ) ;
#18111=VERTEX_POINT ( 'NONE', #6667 ) ;
#18125=CARTESIAN_POINT ( 'NONE',  ( -18.18961309330695997, 35.81157980123359863, -25.80119252674831998 ) ) ;
#18130=EDGE_LOOP ( 'NONE', ( #952, #18983, #3632, #3046 ) ) ;
#18142=EDGE_CURVE ( 'NONE', #6968, #6063, #6698, .T. ) ;
#18143=AXIS2_PLACEMENT_3D ( 'NONE', #2201, #12599, #14056 ) ;
#18144=PLANE ( 'NONE',  #5265 ) ;
#18146=CARTESIAN_POINT ( 'NONE',  ( 11.42842559562532578, -3.968114999999999615, 1.673196738795719174 ) ) ;
#18164=VECTOR ( 'NONE', #16252, 1000.000000000000000 ) ;
#18170=DIRECTION ( 'NONE',  ( -0.9685006480810793850, 0.000000000000000000, -0.2490110332224846623 ) ) ;
#18174=VECTOR ( 'NONE', #18374, 1000.000000000000000 ) ;
#18188=DIRECTION ( 'NONE',  ( 0.000000000000000000, 1.000000000000000000, 0.000000000000000000 ) ) ;
#18200=EDGE_CURVE ( 'NONE', #1715, #13378, #7644, .T. ) ;
#18211=DIRECTION ( 'NONE',  ( -0.000000000000000000, -1.000000000000000000, 0.000000000000000000 ) ) ;
#18212=ORIENTED_EDGE ( 'NONE', *, *, #1837, .T. ) ;
#18216=VERTEX_POINT ( 'NONE', #18146 ) ;
#18224=DIRECTION ( 'NONE',  ( -0.2672484743474505819, 0.000000000000000000, -0.9636276526537416176 ) ) ;
#18232=DIRECTION ( 'NONE',  ( -0.08420877549337302259, 0.000000000000000000, -0.9964481331860212121 ) ) ;
#18242=CARTESIAN_POINT ( 'NONE',  ( 59.61686353177688602, -3.968114999999999615, -0.7993558564620834028 ) ) ;
#18252=EDGE_LOOP ( 'NONE', ( #7612, #1122, #8448, #2129 ) ) ;
#18256=ORIENTED_EDGE ( 'NONE', *, *, #18024, .F. ) ;
#18258=LINE ( 'NONE', #14755, #5252 ) ;
#18264=EDGE_CURVE ( 'NONE', #17843, #20607, #8113, .T. ) ;
#18270=DIRECTION ( 'NONE',  ( 0.000000000000000000, 1.000000000000000000, 0.000000000000000000 ) ) ;
#18274=DIRECTION ( 'NONE',  ( -0.000000000000000000, -1.000000000000000000, 0.000000000000000000 ) ) ;
#18276=LINE ( 'NONE', #13223, #12827 ) ;
#18280=ORIENTED_EDGE ( 'NONE', *, *, #19262, .T. ) ;
#18282=CARTESIAN_POINT ( 'NONE',  ( 17.99520596118501814, -14.84248999999999974, -14.84645223781840073 ) ) ;
#18285=CARTESIAN_POINT ( 'NONE',  ( 59.61686353177688602, -1.983739999999999393, -0.7993558564620834028 ) ) ;
#18291=ORIENTED_EDGE ( 'NONE', *, *, #13685, .T. ) ;
#18292=ADVANCED_FACE ( 'NONE', ( #19675 ), #4220, .T. ) ;
#18301=VERTEX_POINT ( 'NONE', #4335 ) ;
#18307=ORIENTED_EDGE ( 'NONE', *, *, #12203, .F. ) ;
#18309=AXIS2_PLACEMENT_3D ( 'NONE', #18828, #5338, #12103 ) ;
#18312=CARTESIAN_POINT ( 'NONE',  ( -16.73439918454169018, 37.15413452960619622, -25.92417111164088084 ) ) ;
#18316=ORIENTED_EDGE ( 'NONE', *, *, #3132, .T. ) ;
#18319=EDGE_LOOP ( 'NONE', ( #16528, #11167, #12023, #6243, #7979, #14257 ) ) ;
#18322=FACE_OUTER_BOUND ( 'NONE', #2057, .T. ) ;
#18353=FACE_OUTER_BOUND ( 'NONE', #21194, .T. ) ;
#18370=CARTESIAN_POINT ( 'NONE',  ( 12.13621795668766445, -1.983739999999999393, 4.225309685850866082 ) ) ;
#18374=DIRECTION ( 'NONE',  ( 0.08420877549337300871, 0.000000000000000000, 0.9964481331860212121 ) ) ;
#18378=PLANE ( 'NONE',  #1079 ) ;
#18379=EDGE_CURVE ( 'NONE', #4031, #19334, #18618, .T. ) ;
#18388=CYLINDRICAL_SURFACE ( 'NONE', #17708, 1.983740000000000281 ) ;
#18391=CARTESIAN_POINT ( 'NONE',  ( 2.915917464538113180, 34.52875999999999834, -18.72348548116188027 ) ) ;
#18408=ORIENTED_EDGE ( 'NONE', *, *, #11699, .F. ) ;
#18409=EDGE_CURVE ( 'NONE', #15141, #9888, #12243, .T. ) ;
#18413=DIRECTION ( 'NONE',  ( -0.08420877549337300871, 0.000000000000000000, -0.9964481331860212121 ) ) ;
#18418=FACE_OUTER_BOUND ( 'NONE', #9879, .T. ) ;
#18425=EDGE_LOOP ( 'NONE', ( #6488, #3852, #19447, #21329 ) ) ;
#18444=ORIENTED_EDGE ( 'NONE', *, *, #4372, .F. ) ;
#18449=VERTEX_POINT ( 'NONE', #3841 ) ;
#18453=AXIS2_PLACEMENT_3D ( 'NONE', #13493, #10157, #8609 ) ;
#18454=AXIS2_PLACEMENT_3D ( 'NONE', #16931, #13317, #15088 ) ;
#18469=CARTESIAN_POINT ( 'NONE',  ( 29.01020070778135818, 36.51313500000000545, -13.85841188422236492 ) ) ;
#18480=EDGE_CURVE ( 'NONE', #4038, #9564, #12378, .T. ) ;
#18494=CARTESIAN_POINT ( 'NONE',  ( 11.56192577415882816, -1.983739999999999393, 4.677561850332325299 ) ) ;
#18500=EDGE_LOOP ( 'NONE', ( #8340, #14286 ) ) ;
#18515=CIRCLE ( 'NONE', #5106, 0.7950200000000000600 ) ;
#18516=EDGE_CURVE ( 'NONE', #9986, #13702, #6364, .T. ) ;
#18525=ORIENTED_EDGE ( 'NONE', *, *, #6926, .T. ) ;
#18543=ORIENTED_EDGE ( 'NONE', *, *, #11172, .F. ) ;
#18550=EDGE_LOOP ( 'NONE', ( #21478, #17097, #13298, #16227 ) ) ;
#18569=LINE ( 'NONE', #10064, #12428 ) ;
#18578=EDGE_CURVE ( 'NONE', #18301, #7937, #14088, .T. ) ;
#18584=DIRECTION ( 'NONE',  ( 0.9964481331860212121, 0.000000000000000000, -0.08420877549337300871 ) ) ;
#18587=CARTESIAN_POINT ( 'NONE',  ( 17.87574706213523612, 34.52875999999999834, -11.18912023382283571 ) ) ;
#18592=CARTESIAN_POINT ( 'NONE',  ( 17.22522857595987844, -3.968114999999999615, -15.04442098945225403 ) ) ;
#18618=( BOUNDED_CURVE ( )  B_SPLINE_CURVE ( 3, ( #18864, #11810, #1730, #18967 ),
 .UNSPECIFIED., .F., .F. ) 
 B_SPLINE_CURVE_WITH_KNOTS ( ( 4, 4 ),
 ( 4.712388980384379700, 5.083959002914050451 ),
 .UNSPECIFIED. ) 
 CURVE ( )  GEOMETRIC_REPRESENTATION_ITEM ( )  RATIONAL_B_SPLINE_CURVE ( ( 1.000000000000000000, 0.9885276984536621736, 0.9885276984536621736, 1.000000000000000000 ) ) 
 REPRESENTATION_ITEM ( '' )  );
#18631=DIRECTION ( 'NONE',  ( 0.08420877549337300871, 0.000000000000000000, 0.9964481331860212121 ) ) ;
#18632=AXIS2_PLACEMENT_3D ( 'NONE', #14296, #10948, #17260 ) ;
#18633=VERTEX_POINT ( 'NONE', #21027 ) ;
#18635=ORIENTED_EDGE ( 'NONE', *, *, #12589, .F. ) ;
#18644=CARTESIAN_POINT ( 'NONE',  ( 19.79515554403045741, 36.51313500000000545, -10.69562145279641996 ) ) ;
#18654=CARTESIAN_POINT ( 'NONE',  ( 9.907371917564091746, 34.52875999999999834, -13.23786778167655243 ) ) ;
#18660=VECTOR ( 'NONE', #20198, 1000.000000000000114 ) ;
#18661=ADVANCED_FACE ( 'NONE', ( #12533 ), #800, .F. ) ;
#18662=AXIS2_PLACEMENT_3D ( 'NONE', #694, #9421, #16194 ) ;
#18671=ORIENTED_EDGE ( 'NONE', *, *, #149, .T. ) ;
#18676=ADVANCED_FACE ( 'NONE', ( #10526 ), #4013, .T. ) ;
#18681=CARTESIAN_POINT ( 'NONE',  ( -16.07247711516169275, -2.588178535606159958, -10.44681224123558039 ) ) ;
#18682=CIRCLE ( 'NONE', #14836, 0.7950200000000003930 ) ;
#18686=VECTOR ( 'NONE', #6554, 1000.000000000000000 ) ;
#18700=DIRECTION ( 'NONE',  ( -0.9964481331860212121, 0.000000000000000000, 0.08420877549337305035 ) ) ;
#18707=CARTESIAN_POINT ( 'NONE',  ( 14.25617145423489696, 36.51313500000000545, -15.80779474975094168 ) ) ;
#18714=LINE ( 'NONE', #10208, #9562 ) ;
#18731=EDGE_LOOP ( 'NONE', ( #870, #17034, #18444, #714 ) ) ;
#18743=VERTEX_POINT ( 'NONE', #2682 ) ;
#18752=LINE ( 'NONE', #15248, #8658 ) ;
#18760=LINE ( 'NONE', #5385, #9502 ) ;
#18763=ORIENTED_EDGE ( 'NONE', *, *, #3508, .T. ) ;
#18767=ORIENTED_EDGE ( 'NONE', *, *, #4298, .T. ) ;
#18776=AXIS2_PLACEMENT_3D ( 'NONE', #8591, #16997, #21651 ) ;
#18779=CYLINDRICAL_SURFACE ( 'NONE', #2287, 1.191259999999998209 ) ;
#18783=CARTESIAN_POINT ( 'NONE',  ( -51.02421882195815783, 38.25938500000000175, -23.02637480153789795 ) ) ;
#18787=ORIENTED_EDGE ( 'NONE', *, *, #4494, .F. ) ;
#18792=DIRECTION ( 'NONE',  ( -0.9685006480810794960, 0.000000000000000000, -0.2490110332224836354 ) ) ;
#18794=DIRECTION ( 'NONE',  ( 0.000000000000000000, 1.000000000000000000, 0.000000000000000000 ) ) ;
#18802=VECTOR ( 'NONE', #5262, 1000.000000000000000 ) ;
#18808=CARTESIAN_POINT ( 'NONE',  ( -22.90765545213488963, -6.903720000000000745, -9.869178565316103047 ) ) ;
#18818=LINE ( 'NONE', #3686, #15083 ) ;
#18822=CARTESIAN_POINT ( 'NONE',  ( 22.02657784715807665, 34.52875999999999834, -12.98906981665815330 ) ) ;
#18828=CARTESIAN_POINT ( 'NONE',  ( -24.20935654380574320, -6.905625000000000568, -25.29247038871795894 ) ) ;
#18831=EDGE_LOOP ( 'NONE', ( #15926, #14368, #8049, #2489 ) ) ;
#18841=LINE ( 'NONE', #10450, #17662 ) ;
#18846=EDGE_LOOP ( 'NONE', ( #14334, #19991, #10624, #2281 ) ) ;
#18855=AXIS2_PLACEMENT_3D ( 'NONE', #4847, #4743, #7250 ) ;
#18864=CARTESIAN_POINT ( 'NONE',  ( -13.87568970999206108, -1.983739999999999393, -9.457638332870221376 ) ) ;
#18866=CARTESIAN_POINT ( 'NONE',  ( 12.25799425556778388, 36.51313500000000545, 0.2069032437451798767 ) ) ;
#18872=FILL_AREA_STYLE ('',( #8592 ) ) ;
#18875=ORIENTED_EDGE ( 'NONE', *, *, #16116, .T. ) ;
#18882=ORIENTED_EDGE ( 'NONE', *, *, #21103, .F. ) ;
#18896=DIRECTION ( 'NONE',  ( -0.9964481331860213231, 0.000000000000000000, 0.08420877549337293932 ) ) ;
#18921=CYLINDRICAL_SURFACE ( 'NONE', #12933, 20.83593749999999289 ) ;
#18929=EDGE_CURVE ( 'NONE', #3364, #9466, #16912, .T. ) ;
#18934=DIRECTION ( 'NONE',  ( 0.9685006480810793850, 0.000000000000000000, 0.2490110332224846623 ) ) ;
#18946=ORIENTED_EDGE ( 'NONE', *, *, #2345, .T. ) ;
#18949=ORIENTED_EDGE ( 'NONE', *, *, #15365, .F. ) ;
#18950=EDGE_CURVE ( 'NONE', #8103, #21087, #9832, .T. ) ;
#18952=LINE ( 'NONE', #9552, #2853 ) ;
#18953=DIRECTION ( 'NONE',  ( 0.000000000000000000, 1.000000000000000000, 0.000000000000000000 ) ) ;
#18956=DIRECTION ( 'NONE',  ( 0.000000000000000000, 1.000000000000000000, 0.000000000000000000 ) ) ;
#18965=CARTESIAN_POINT ( 'NONE',  ( 3.360635606688116894, 36.51313500000000545, -20.45316710734507026 ) ) ;
#18967=CARTESIAN_POINT ( 'NONE',  ( -15.39353573898878658, -2.254660308866960339, -10.30107656633069979 ) ) ;
#18976=CARTESIAN_POINT ( 'NONE',  ( 14.25617145423489696, 34.52875999999999834, -15.80779474975094168 ) ) ;
#18982=CYLINDRICAL_SURFACE ( 'NONE', #4670, 3.970019999999997662 ) ;
#18983=ORIENTED_EDGE ( 'NONE', *, *, #19891, .T. ) ;
#18991=AXIS2_PLACEMENT_3D ( 'NONE', #17313, #283, #2040 ) ;
#19001=LINE ( 'NONE', #12391, #13485 ) ;
#19003=CARTESIAN_POINT ( 'NONE',  ( 11.82678039945931481, -1.983739999999999393, -12.74436900065013667 ) ) ;
#19025=AXIS2_PLACEMENT_3D ( 'NONE', #21867, #6282, #4525 ) ;
#19029=CARTESIAN_POINT ( 'NONE',  ( 46.03750000000000142, -14.84248999999999974, -10.31874999999999964 ) ) ;
#19031=CYLINDRICAL_SURFACE ( 'NONE', #8506, 0.7950200000000000600 ) ;
#19032=AXIS2_PLACEMENT_3D ( 'NONE', #1392, #13255, #8134 ) ;
#19036=CARTESIAN_POINT ( 'NONE',  ( 12.79472653632228507, -3.968114999999999615, -13.31637763425449883 ) ) ;
#19040=PRODUCT_CONTEXT ( 'NONE', #20604, 'mechanical' ) ;
#19043=PRODUCT_DEFINITION_SHAPE ( 'NONE', 'NONE',  #471 ) ;
#19051=DIRECTION ( 'NONE',  ( -0.2490110332224848011, 0.000000000000000000, 0.9685006480810792739 ) ) ;
#19054=VECTOR ( 'NONE', #10740, 1000.000000000000114 ) ;
#19058=CARTESIAN_POINT ( 'NONE',  ( 12.25799425556778388, -1.983739999999999393, 0.2069032437451798767 ) ) ;
#19059=EDGE_LOOP ( 'NONE', ( #19968, #12541, #5366, #7838 ) ) ;
#19065=DIRECTION ( 'NONE',  ( 0.000000000000000000, 1.000000000000000000, 0.000000000000000000 ) ) ;
#19068=VECTOR ( 'NONE', #15337, 1000.000000000000000 ) ;
#19070=LINE ( 'NONE', #9345, #3675 ) ;
#19071=EDGE_CURVE ( 'NONE', #6701, #5934, #3107, .T. ) ;
#19079=AXIS2_PLACEMENT_3D ( 'NONE', #14674, #9223, #4261 ) ;
#19088=CARTESIAN_POINT ( 'NONE',  ( -15.27766260488554195, 38.49878000000000355, -26.04727837583638461 ) ) ;
#19089=VECTOR ( 'NONE', #487, 1000.000000000000114 ) ;
#19092=AXIS2_PLACEMENT_3D ( 'NONE', #14801, #6367, #18211 ) ;
#19096=ORIENTED_EDGE ( 'NONE', *, *, #18578, .F. ) ;
#19103=ORIENTED_EDGE ( 'NONE', *, *, #3116, .F. ) ;
#19106=EDGE_CURVE ( 'NONE', #9783, #20277, #18569, .T. ) ;
#19110=DIRECTION ( 'NONE',  ( 0.9685006480810793850, 0.000000000000000000, 0.2490110332224846623 ) ) ;
#19112=VECTOR ( 'NONE', #1759, 1000.000000000000000 ) ;
#19133=ADVANCED_FACE ( 'NONE', ( #1652 ), #8393, .T. ) ;
#19137=EDGE_CURVE ( 'NONE', #9564, #13936, #4088, .T. ) ;
#19140=CARTESIAN_POINT ( 'NONE',  ( 17.30373842852263877, 34.52875999999999834, -12.15706637069277107 ) ) ;
#19162=DIRECTION ( 'NONE',  ( 0.9964481331860213231, 0.000000000000000000, -0.08420877549337293932 ) ) ;
#19172=CARTESIAN_POINT ( 'NONE',  ( 29.01020070778135818, -1.983739999999999393, -13.85841188422236492 ) ) ;
#19180=DIRECTION ( 'NONE',  ( 0.08420877549337300871, 0.000000000000000000, 0.9964481331860212121 ) ) ;
#19187=EDGE_CURVE ( 'NONE', #7846, #7070, #5407, .T. ) ;
#19199=DIRECTION ( 'NONE',  ( 0.2490110332224846623, 0.000000000000000000, -0.9685006480810793850 ) ) ;
#19202=CARTESIAN_POINT ( 'NONE',  ( 17.30373842852263877, 36.51313500000000545, -12.15706637069277107 ) ) ;
#19204=AXIS2_PLACEMENT_3D ( 'NONE', #4445, #12858, #16174 ) ;
#19207=CARTESIAN_POINT ( 'NONE',  ( 2.915917464538113180, -1.983739999999999393, -18.72348548116188027 ) ) ;
#19214=VECTOR ( 'NONE', #4567, 1000.000000000000000 ) ;
#19228=DIRECTION ( 'NONE',  ( -0.000000000000000000, -1.000000000000000000, 0.000000000000000000 ) ) ;
#19233=VERTEX_POINT ( 'NONE', #5517 ) ;
#19252=CARTESIAN_POINT ( 'NONE',  ( -15.39353573898878658, 37.13217763270220217, -10.30107656633069979 ) ) ;
#19255=FACE_OUTER_BOUND ( 'NONE', #12064, .T. ) ;
#19260=EDGE_CURVE ( 'NONE', #13482, #10479, #6760, .T. ) ;
#19262=EDGE_CURVE ( 'NONE', #8566, #19617, #19001, .T. ) ;
#19268=DIRECTION ( 'NONE',  ( -0.000000000000000000, -1.000000000000000000, 0.000000000000000000 ) ) ;
#19273=VERTEX_POINT ( 'NONE', #3985 ) ;
#19274=CARTESIAN_POINT ( 'NONE',  ( 10.10534066920194185, 34.52875999999999834, -14.00784516691476966 ) ) ;
#19290=CARTESIAN_POINT ( 'NONE',  ( -15.39353573898878658, 34.79968030885680008, -10.30107656633069979 ) ) ;
#19293=DIRECTION ( 'NONE',  ( -0.9685006480810794960, 0.000000000000000000, -0.2490110332224836354 ) ) ;
#19304=FACE_OUTER_BOUND ( 'NONE', #1824, .T. ) ;
#19306=CARTESIAN_POINT ( 'NONE',  ( -15.27766260488554195, -1.983739999999999393, -26.04727837583638461 ) ) ;
#19312=VERTEX_POINT ( 'NONE', #18783 ) ;
#19315=CARTESIAN_POINT ( 'NONE',  ( 17.79723720954694954, 36.51313500000000545, -14.07647485258271303 ) ) ;
#19320=EDGE_LOOP ( 'NONE', ( #6707, #18946, #11904, #605 ) ) ;
#19322=CARTESIAN_POINT ( 'NONE',  ( -22.47451353405102026, 43.41875999999999891, -25.43908013252627853 ) ) ;
#19332=CARTESIAN_POINT ( 'NONE',  ( 29.01020070778135818, 34.52875999999999834, -13.85841188422236492 ) ) ;
#19334=VERTEX_POINT ( 'NONE', #9599 ) ;
#19336=CARTESIAN_POINT ( 'NONE',  ( 46.03750000000000142, 36.51313500000000545, -10.31874999999999964 ) ) ;
#19346=CIRCLE ( 'NONE', #9808, 1.983740000000000059 ) ;
#19348=CARTESIAN_POINT ( 'NONE',  ( 9.335363283976800375, -1.983739999999999393, -14.20581391854862474 ) ) ;
#19351=LINE ( 'NONE', #21777, #19407 ) ;
#19352=LINE ( 'NONE', #12528, #20232 ) ;
#19357=EDGE_CURVE ( 'NONE', #5833, #16351, #13150, .T. ) ;
#19364=ORIENTED_EDGE ( 'NONE', *, *, #17833, .T. ) ;
#19366=VECTOR ( 'NONE', #16816, 1000.000000000000000 ) ;
#19368=EDGE_LOOP ( 'NONE', ( #1860, #428, #4929, #15498 ) ) ;
#19374=DIRECTION ( 'NONE',  ( 0.000000000000000000, 1.000000000000000000, 0.000000000000000000 ) ) ;
#19379=VECTOR ( 'NONE', #19762, 1000.000000000000000 ) ;
#19397=CARTESIAN_POINT ( 'NONE',  ( 12.57635667311951622, 34.52875999999999834, 1.354834321244424267 ) ) ;
#19407=VECTOR ( 'NONE', #8389, 1000.000000000000000 ) ;
#19408=LINE ( 'NONE', #19306, #1314 ) ;
#19412=AXIS2_PLACEMENT_3D ( 'NONE', #4922, #11563, #7919 ) ;
#19419=DIRECTION ( 'NONE',  ( -0.2490110332224846346, 0.000000000000000000, 0.9685006480810792739 ) ) ;
#19430=CYLINDRICAL_SURFACE ( 'NONE', #2630, 1.785937499999999512 ) ;
#19433=CYLINDRICAL_SURFACE ( 'NONE', #17484, 0.7950200000000000600 ) ;
#19438=DIRECTION ( 'NONE',  ( 0.000000000000000000, 1.000000000000000000, 0.000000000000000000 ) ) ;
#19447=ORIENTED_EDGE ( 'NONE', *, *, #19488, .F. ) ;
#19449=VERTEX_POINT ( 'NONE', #2984 ) ;
#19450=CARTESIAN_POINT ( 'NONE',  ( 17.87574706213523612, -1.983739999999999393, -11.18912023382283571 ) ) ;
#19477=ORIENTED_EDGE ( 'NONE', *, *, #9369, .T. ) ;
#19488=EDGE_CURVE ( 'NONE', #17560, #3364, #15630, .T. ) ;
#19490=VECTOR ( 'NONE', #11253, 1000.000000000000000 ) ;
#19496=CARTESIAN_POINT ( 'NONE',  ( 29.45491884992628329, -3.968114999999999615, -15.58809351040512325 ) ) ;
#19498=AXIS2_PLACEMENT_3D ( 'NONE', #14491, #19657, #2868 ) ;
#19507=DIRECTION ( 'NONE',  ( 0.000000000000000000, 1.000000000000000000, 0.000000000000000000 ) ) ;
#19514=CARTESIAN_POINT ( 'NONE',  ( 14.25617145423489696, -1.983739999999999393, -15.80779474975094168 ) ) ;
#19515=ORIENTED_EDGE ( 'NONE', *, *, #1905, .F. ) ;
#19527=AXIS2_PLACEMENT_3D ( 'NONE', #5975, #4338, #17834 ) ;
#19529=DIRECTION ( 'NONE',  ( 0.9964481331860213231, 0.000000000000000000, -0.08420877549337293932 ) ) ;
#19532=CYLINDRICAL_SURFACE ( 'NONE', #7188, 0.3962400000000000366 ) ;
#19535=CARTESIAN_POINT ( 'NONE',  ( -15.71080452296940599, -14.84248999999999974, -10.47737680862620380 ) ) ;
#19539=EDGE_CURVE ( 'NONE', #8727, #20432, #15993, .T. ) ;
#19542=CARTESIAN_POINT ( 'NONE',  ( 22.22454659879084460, 34.52875999999999834, -13.75904720189594244 ) ) ;
#19550=AXIS2_PLACEMENT_3D ( 'NONE', #16595, #8496, #11724 ) ;
#19561=EDGE_CURVE ( 'NONE', #14476, #12395, #81, .T. ) ;
#19562=ORIENTED_EDGE ( 'NONE', *, *, #14720, .F. ) ;
#19569=EDGE_LOOP ( 'NONE', ( #15124, #1274, #1961, #11266 ) ) ;
#19576=DIRECTION ( 'NONE',  ( -0.9964481331860212121, 0.000000000000000000, 0.08420877549337336954 ) ) ;
#19588=CARTESIAN_POINT ( 'NONE',  ( -46.55773479047372376, 43.41875999999999891, -7.870535429687039120 ) ) ;
#19600=CIRCLE ( 'NONE', #1944, 9.525000000000002132 ) ;
#19606=DIRECTION ( 'NONE',  ( 0.08420877549337300871, 0.000000000000000000, 0.9964481331860212121 ) ) ;
#19610=DIRECTION ( 'NONE',  ( 0.000000000000000000, 1.000000000000000000, 0.000000000000000000 ) ) ;
#19612=ORIENTED_EDGE ( 'NONE', *, *, #212, .F. ) ;
#19617=VERTEX_POINT ( 'NONE', #20294 ) ;
#19622=ORIENTED_EDGE ( 'NONE', *, *, #8817, .F. ) ;
#19624=EDGE_CURVE ( 'NONE', #12588, #11891, #4852, .T. ) ;
#19629=ORIENTED_EDGE ( 'NONE', *, *, #10715, .T. ) ;
#19641=ORIENTED_EDGE ( 'NONE', *, *, #13685, .F. ) ;
#19649=LINE ( 'NONE', #2647, #20252 ) ;
#19654=DIRECTION ( 'NONE',  ( -0.9685006480810792739, 0.000000000000000000, -0.2490110332224846346 ) ) ;
#19657=DIRECTION ( 'NONE',  ( 0.000000000000000000, 1.000000000000000000, 0.000000000000000000 ) ) ;
#19659=ORIENTED_EDGE ( 'NONE', *, *, #5454, .F. ) ;
#19662=CARTESIAN_POINT ( 'NONE',  ( 17.30373842852263877, 34.52875999999999834, -12.15706637069277107 ) ) ;
#19675=FACE_OUTER_BOUND ( 'NONE', #276, .T. ) ;
#19694=CARTESIAN_POINT ( 'NONE',  ( 12.25799425556778388, 36.51313500000000545, 0.2069032437451798767 ) ) ;
#19705=FACE_BOUND ( 'NONE', #16052, .T. ) ;
#19706=DIRECTION ( 'NONE',  ( -0.9964481331860212121, 0.000000000000000000, 0.08420877549337300871 ) ) ;
#19708=CARTESIAN_POINT ( 'NONE',  ( -22.75431282566211522, 40.79338547039380103, -25.41543459098148716 ) ) ;
#19719=VECTOR ( 'NONE', #9814, 1000.000000000000000 ) ;
#19732=DIRECTION ( 'NONE',  ( 0.2490110332224848289, 0.000000000000000000, -0.9685006480810792739 ) ) ;
#19742=EDGE_CURVE ( 'NONE', #13996, #7176, #16887, .T. ) ;
#19744=ORIENTED_EDGE ( 'NONE', *, *, #8812, .T. ) ;
#19745=ADVANCED_FACE ( 'NONE', ( #14148 ), #13808, .F. ) ;
#19747=EDGE_CURVE ( 'NONE', #6259, #10166, #10369, .T. ) ;
#19750=AXIS2_PLACEMENT_3D ( 'NONE', #16175, #2775, #21338 ) ;
#19754=CARTESIAN_POINT ( 'NONE',  ( 46.03750000000000142, -14.84248999999999974, -10.31874999999999964 ) ) ;
#19757=EDGE_LOOP ( 'NONE', ( #2783, #18408, #10501, #3640 ) ) ;
#19758=PLANE ( 'NONE',  #10713 ) ;
#19760=CARTESIAN_POINT ( 'NONE',  ( 19.79515554403045741, 34.52875999999999834, -10.69562145279641996 ) ) ;
#19762=DIRECTION ( 'NONE',  ( 0.000000000000000000, 1.000000000000000000, 0.000000000000000000 ) ) ;
#19763=ORIENTED_EDGE ( 'NONE', *, *, #10351, .T. ) ;
#19766=APPLICATION_CONTEXT ( 'automotive_design' ) ;
#19768=VERTEX_POINT ( 'NONE', #12248 ) ;
#19778=AXIS2_PLACEMENT_3D ( 'NONE', #15809, #7604, #6163 ) ;
#19785=ORIENTED_EDGE ( 'NONE', *, *, #4219, .T. ) ;
#19794=VERTEX_POINT ( 'NONE', #5723 ) ;
#19820=FACE_OUTER_BOUND ( 'NONE', #6600, .T. ) ;
#19824=DIRECTION ( 'NONE',  ( 0.000000000000000000, -1.000000000000000000, 0.000000000000000000 ) ) ;
#19840=VERTEX_POINT ( 'NONE', #2706 ) ;
#19850=LINE ( 'NONE', #8025, #742 ) ;
#19853=EDGE_CURVE ( 'NONE', #17882, #20691, #21601, .T. ) ;
#19855=PLANE ( 'NONE',  #19032 ) ;
#19861=ORIENTED_EDGE ( 'NONE', *, *, #10826, .F. ) ;
#19868=DIRECTION ( 'NONE',  ( 0.000000000000000000, 1.000000000000000000, 0.000000000000000000 ) ) ;
#19869=CARTESIAN_POINT ( 'NONE',  ( 28.56548256563643662, -3.968114999999999615, -12.12873025803960658 ) ) ;
#19873=FACE_OUTER_BOUND ( 'NONE', #12811, .T. ) ;
#19883=CARTESIAN_POINT ( 'NONE',  ( 44.28293121686854761, 34.52875999999999834, -31.08068102505560759 ) ) ;
#19891=EDGE_CURVE ( 'NONE', #6728, #12014, #10702, .T. ) ;
#19903=DIRECTION ( 'NONE',  ( 0.08420877549337302259, 0.000000000000000000, 0.9964481331860212121 ) ) ;
#19911=ORIENTED_EDGE ( 'NONE', *, *, #1924, .F. ) ;
#19916=CARTESIAN_POINT ( 'NONE',  ( 13.28822531734660828, 36.51313500000000545, -15.23578611614444078 ) ) ;
#19926=ADVANCED_FACE ( 'NONE', ( #16525 ), #14551, .F. ) ;
#19931=DIRECTION ( 'NONE',  ( -0.000000000000000000, -1.000000000000000000, 0.000000000000000000 ) ) ;
#19935=VERTEX_POINT ( 'NONE', #11322 ) ;
#19952=DIRECTION ( 'NONE',  ( 0.000000000000000000, 1.000000000000000000, 0.000000000000000000 ) ) ;
#19968=ORIENTED_EDGE ( 'NONE', *, *, #21825, .T. ) ;
#19973=EDGE_CURVE ( 'NONE', #9581, #20489, #1846, .T. ) ;
#19981=CARTESIAN_POINT ( 'NONE',  ( 28.56548256563643662, -1.983739999999999393, -12.12873025803960658 ) ) ;
#19983=DIRECTION ( 'NONE',  ( -0.9964481331860212121, 0.000000000000000000, 0.08420877549337302259 ) ) ;
#19984=EDGE_LOOP ( 'NONE', ( #9452, #9192, #19763, #11949 ) ) ;
#19985=EDGE_LOOP ( 'NONE', ( #6425, #3385, #11686, #5077 ) ) ;
#19988=ORIENTED_EDGE ( 'NONE', *, *, #17775, .F. ) ;
#19991=ORIENTED_EDGE ( 'NONE', *, *, #8866, .T. ) ;
#19999=AXIS2_PLACEMENT_3D ( 'NONE', #14880, #19610, #1155 ) ;
#20011=CARTESIAN_POINT ( 'NONE',  ( 11.56192577415882816, 36.51313500000000545, 4.677561850332325299 ) ) ;
#20013=EDGE_CURVE ( 'NONE', #4038, #5560, #14878, .T. ) ;
#20016=EDGE_CURVE ( 'NONE', #15970, #17229, #18276, .T. ) ;
#20017=DIRECTION ( 'NONE',  ( 0.2490110332224846346, 0.000000000000000000, -0.9685006480810792739 ) ) ;
#20026=DIRECTION ( 'NONE',  ( 0.000000000000000000, 1.000000000000000000, 0.000000000000000000 ) ) ;
#20028=AXIS2_PLACEMENT_3D ( 'NONE', #8615, #3874, #7068 ) ;
#20029=ORIENTED_EDGE ( 'NONE', *, *, #5473, .F. ) ;
#20031=VERTEX_POINT ( 'NONE', #11645 ) ;
#20036=ORIENTED_EDGE ( 'NONE', *, *, #8412, .T. ) ;
#20038=EDGE_CURVE ( 'NONE', #16397, #1525, #14668, .T. ) ;
#20043=CIRCLE ( 'NONE', #18632, 3.970019999999998550 ) ;
#20049=CARTESIAN_POINT ( 'NONE',  ( 12.25799425556778388, -1.983739999999999393, 0.2069032437451798767 ) ) ;
#20069=VERTEX_POINT ( 'NONE', #3683 ) ;
#20075=AXIS2_PLACEMENT_3D ( 'NONE', #10252, #16999, #6937 ) ;
#20095=ORIENTED_EDGE ( 'NONE', *, *, #13178, .T. ) ;
#20098=CARTESIAN_POINT ( 'NONE',  ( 31.83819605565793509, 34.52875999999999834, -4.158220719828246814 ) ) ;
#20104=CARTESIAN_POINT ( 'NONE',  ( 9.256853431388732290, -1.983739999999999393, -17.09316853730597074 ) ) ;
#20118=CARTESIAN_POINT ( 'NONE',  ( -16.07247711516169275, 35.13319853559599437, -10.44681224123558039 ) ) ;
#20122=VECTOR ( 'NONE', #19706, 1000.000000000000000 ) ;
#20133=AXIS2_PLACEMENT_3D ( 'NONE', #14365, #2635, #17788 ) ;
#20136=EDGE_CURVE ( 'NONE', #9564, #9371, #15095, .T. ) ;
#20139=DIRECTION ( 'NONE',  ( 0.9685006480810794960, 0.000000000000000000, 0.2490110332224836354 ) ) ;
#20167=AXIS2_PLACEMENT_3D ( 'NONE', #561, #2214, #5413 ) ;
#20170=EDGE_CURVE ( 'NONE', #7176, #11404, #7508, .T. ) ;
#20181=ORIENTED_EDGE ( 'NONE', *, *, #19624, .F. ) ;
#20198=DIRECTION ( 'NONE',  ( 0.9685006480810792739, 0.000000000000000000, 0.2490110332224846346 ) ) ;
#20200=ORIENTED_EDGE ( 'NONE', *, *, #4422, .F. ) ;
#20221=CARTESIAN_POINT ( 'NONE',  ( -23.34164412188400561, -8.889364999999999739, -25.36579984571316615 ) ) ;
#20230=CARTESIAN_POINT ( 'NONE',  ( 31.83819605565793509, 36.51313500000000545, -4.158220719828246814 ) ) ;
#20232=VECTOR ( 'NONE', #16072, 1000.000000000000114 ) ;
#20240=DIRECTION ( 'NONE',  ( 0.9685006480810794960, 0.000000000000000000, 0.2490110332224836354 ) ) ;
#20244=DIRECTION ( 'NONE',  ( 0.08420877549337302259, 0.000000000000000000, 0.9964481331860212121 ) ) ;
#20245=ORIENTED_EDGE ( 'NONE', *, *, #882, .F. ) ;
#20252=VECTOR ( 'NONE', #4517, 1000.000000000000000 ) ;
#20273=DIRECTION ( 'NONE',  ( 0.08420877549337300871, 0.000000000000000000, 0.9964481331860212121 ) ) ;
#20277=VERTEX_POINT ( 'NONE', #612 ) ;
#20279=CARTESIAN_POINT ( 'NONE',  ( 11.82678039945931481, -1.983739999999999393, -12.74436900065013667 ) ) ;
#20287=DIRECTION ( 'NONE',  ( 0.2490110332224836354, 0.000000000000000000, -0.9685006480810794960 ) ) ;
#20288=DIRECTION ( 'NONE',  ( 0.000000000000000000, 1.000000000000000000, 0.000000000000000000 ) ) ;
#20294=CARTESIAN_POINT ( 'NONE',  ( 12.79472653632228507, 36.51313500000000545, -13.31637763425449883 ) ) ;
#20304=ORIENTED_EDGE ( 'NONE', *, *, #6271, .T. ) ;
#20308=ORIENTED_EDGE ( 'NONE', *, *, #19260, .T. ) ;
#20309=EDGE_CURVE ( 'NONE', #227, #12039, #7146, .T. ) ;
#20320=CARTESIAN_POINT ( 'NONE',  ( 21.25660046192028929, 36.51313500000000545, -13.18703856829094079 ) ) ;
#20321=CARTESIAN_POINT ( 'NONE',  ( -13.87568970999206108, 34.52875999999999834, -9.457638332870221376 ) ) ;
#20326=ORIENTED_EDGE ( 'NONE', *, *, #8788, .T. ) ;
#20327=CARTESIAN_POINT ( 'NONE',  ( 36.54633153140314761, -3.968114999999999615, -9.516661413425623550 ) ) ;
#20332=CARTESIAN_POINT ( 'NONE',  ( 14.05820270259704152, 34.52875999999999834, -15.03781736451272444 ) ) ;
#20334=ADVANCED_FACE ( 'NONE', ( #8899 ), #10345, .F. ) ;
#20335=CARTESIAN_POINT ( 'NONE',  ( -46.55773479047372376, -10.87373999999999974, -7.870535429687039120 ) ) ;
#20345=FACE_OUTER_BOUND ( 'NONE', #20756, .T. ) ;
#20347=CARTESIAN_POINT ( 'NONE',  ( 13.28822531734660828, -1.983739999999999393, -15.23578611614444078 ) ) ;
#20360=EDGE_CURVE ( 'NONE', #10557, #227, #12463, .T. ) ;
#20377=LINE ( 'NONE', #13786, #21195 ) ;
#20381=VERTEX_POINT ( 'NONE', #15679 ) ;
#20388=ORIENTED_EDGE ( 'NONE', *, *, #17673, .T. ) ;
#20397=LINE ( 'NONE', #6513, #18802 ) ;
#20416=LINE ( 'NONE', #17020, #5784 ) ;
#20417=CARTESIAN_POINT ( 'NONE',  ( 30.74535937054756829, -95.96551800000000298, -3.684081112461307317 ) ) ;
#20432=VERTEX_POINT ( 'NONE', #4047 ) ;
#20448=CARTESIAN_POINT ( 'NONE',  ( 11.82678039945931481, 36.51313500000000545, -12.74436900065013667 ) ) ;
#20451=DIRECTION ( 'NONE',  ( -0.7334850928793775759, -0.6768732144311021548, 0.06198604769977036216 ) ) ;
#20453=EDGE_CURVE ( 'NONE', #17468, #11383, #2218, .T. ) ;
#20467=ORIENTED_EDGE ( 'NONE', *, *, #2080, .T. ) ;
#20469=CARTESIAN_POINT ( 'NONE',  ( -15.27935546639805331, 36.51313500000000545, -26.04713531390440906 ) ) ;
#20470=CARTESIAN_POINT ( 'NONE',  ( 62.90077106633562209, 34.52875999999999834, 8.141649473166729933 ) ) ;
#20485=LINE ( 'NONE', #5355, #19068 ) ;
#20489=VERTEX_POINT ( 'NONE', #5081 ) ;
#20497=CIRCLE ( 'NONE', #8153, 9.524999999999996803 ) ;
#20501=LINE ( 'NONE', #5154, #15691 ) ;
#20509=EDGE_CURVE ( 'NONE', #4266, #17362, #21282, .T. ) ;
#20516=DIRECTION ( 'NONE',  ( -0.2490110332224848011, 0.000000000000000000, 0.9685006480810792739 ) ) ;
#20536=DIRECTION ( 'NONE',  ( 0.000000000000000000, 1.000000000000000000, 0.000000000000000000 ) ) ;
#20544=CARTESIAN_POINT ( 'NONE',  ( 30.74535937054756829, 36.51313500000000545, -3.684081112461307317 ) ) ;
#20562=ADVANCED_FACE ( 'NONE', ( #11533 ), #8097, .F. ) ;
#20564=CARTESIAN_POINT ( 'NONE',  ( 18.07371581377308800, -3.968114999999999615, -11.95909761906105473 ) ) ;
#20574=DIRECTION ( 'NONE',  ( 0.9636276526537417286, 0.000000000000000000, -0.2672484743474500268 ) ) ;
#20575=PLANE ( 'NONE',  #17514 ) ;
#20591=ADVANCED_FACE ( 'NONE', ( #2703, #19705, #16626 ), #17960, .F. ) ;
#20600=CARTESIAN_POINT ( 'NONE',  ( 9.335363283976800375, 36.51313500000000545, -14.20581391854862474 ) ) ;
#20604=APPLICATION_CONTEXT ( 'automotive_design' ) ;
#20607=VERTEX_POINT ( 'NONE', #4894 ) ;
#20609=DIRECTION ( 'NONE',  ( -0.7334850928793776870, -0.6768732144311019328, 0.06198604769976998052 ) ) ;
#20614=CARTESIAN_POINT ( 'NONE',  ( -15.97216256926745714, -95.96551800000000298, -9.259783438096400587 ) ) ;
#20615=ORIENTED_EDGE ( 'NONE', *, *, #10848, .F. ) ;
#20624=VECTOR ( 'NONE', #20764, 1000.000000000000000 ) ;
#20628=DIRECTION ( 'NONE',  ( 0.2490110332224846346, 0.000000000000000000, -0.9685006480810792739 ) ) ;
#20631=CARTESIAN_POINT ( 'NONE',  ( 3.805353748838121053, -1.983739999999999393, -22.18284873352824960 ) ) ;
#20644=VECTOR ( 'NONE', #1624, 1000.000000000000000 ) ;
#20650=FACE_OUTER_BOUND ( 'NONE', #12157, .T. ) ;
#20653=DIRECTION ( 'NONE',  ( -0.9685006480810792739, 0.000000000000000000, -0.2490110332224846346 ) ) ;
#20658=CARTESIAN_POINT ( 'NONE',  ( -16.07247711516169275, 35.13319853559599437, -10.44681224123558039 ) ) ;
#20660=DIRECTION ( 'NONE',  ( 0.000000000000000000, 1.000000000000000000, 0.000000000000000000 ) ) ;
#20664=DIRECTION ( 'NONE',  ( 0.000000000000000000, 1.000000000000000000, 0.000000000000000000 ) ) ;
#20676=CYLINDRICAL_SURFACE ( 'NONE', #9150, 0.7950200000000000600 ) ;
#20691=VERTEX_POINT ( 'NONE', #20321 ) ;
#20728=ORIENTED_EDGE ( 'NONE', *, *, #6413, .F. ) ;
#20730=CARTESIAN_POINT ( 'NONE',  ( 12.25799425556778388, -3.968114999999999615, 0.2069032437451798767 ) ) ;
#20734=CARTESIAN_POINT ( 'NONE',  ( -46.55710204590916135, 38.25938500000000175, -7.870588902259476605 ) ) ;
#20739=ORIENTED_EDGE ( 'NONE', *, *, #6125, .T. ) ;
#20743=DIRECTION ( 'NONE',  ( -0.000000000000000000, -1.000000000000000000, 0.000000000000000000 ) ) ;
#20748=EDGE_CURVE ( 'NONE', #8700, #15141, #3218, .T. ) ;
#20756=EDGE_LOOP ( 'NONE', ( #1360, #2064, #8353, #8245, #11945, #16371 ) ) ;
#20759=ORIENTED_EDGE ( 'NONE', *, *, #12330, .F. ) ;
#20760=AXIS2_PLACEMENT_3D ( 'NONE', #20470, #6789, #15326 ) ;
#20764=DIRECTION ( 'NONE',  ( 0.000000000000000000, 1.000000000000000000, 0.000000000000000000 ) ) ;
#20779=CARTESIAN_POINT ( 'NONE',  ( -51.02421882195815783, -5.714364999999999029, -23.02637480153789795 ) ) ;
#20790=LINE ( 'NONE', #15749, #15307 ) ;
#20793=CARTESIAN_POINT ( 'NONE',  ( -23.34164412188400561, 41.43438499999999891, -25.36579984571316615 ) ) ;
#20807=PLANE ( 'NONE',  #2859 ) ;
#20816=DIRECTION ( 'NONE',  ( -0.7334850928793772429, 0.6768732144311025989, 0.06198604769976985562 ) ) ;
#20817=CARTESIAN_POINT ( 'NONE',  ( 9.256853431388732290, -1.983739999999999393, -17.09316853730597074 ) ) ;
#20830=AXIS2_PLACEMENT_3D ( 'NONE', #15966, #20574, #15643 ) ;
#20832=CARTESIAN_POINT ( 'NONE',  ( -51.69815163306579819, -5.714999999999999858, -7.436124251198355850 ) ) ;
#20833=VERTEX_POINT ( 'NONE', #20658 ) ;
#20834=( NAMED_UNIT ( * ) PLANE_ANGLE_UNIT ( ) SI_UNIT ( $, .RADIAN. ) );
#20836=ORIENTED_EDGE ( 'NONE', *, *, #16446, .F. ) ;
#20842=EDGE_CURVE ( 'NONE', #1054, #17145, #12446, .T. ) ;
#20844=AXIS2_PLACEMENT_3D ( 'NONE', #15024, #10125, #172 ) ;
#20850=CARTESIAN_POINT ( 'NONE',  ( 13.28822531734660828, -1.983739999999999393, -15.23578611614444078 ) ) ;
#20854=VECTOR ( 'NONE', #8546, 1000.000000000000000 ) ;
#20855=VERTEX_POINT ( 'NONE', #4197 ) ;
#20859=CARTESIAN_POINT ( 'NONE',  ( 59.61686353177688602, 36.51313500000000545, -0.7993558564620834028 ) ) ;
#20861=VERTEX_POINT ( 'NONE', #17690 ) ;
#20868=AXIS2_PLACEMENT_3D ( 'NONE', #10866, #16403, #14752 ) ;
#20873=DIRECTION ( 'NONE',  ( 0.9636276526537417286, 0.000000000000000000, -0.2672484743474499158 ) ) ;
#20876=VECTOR ( 'NONE', #6630, 1000.000000000000000 ) ;
#20879=DIRECTION ( 'NONE',  ( 0.000000000000000000, 1.000000000000000000, 0.000000000000000000 ) ) ;
#20886=CARTESIAN_POINT ( 'NONE',  ( -16.88621914012359326, -3.266559801243759331, -10.37804376527844141 ) ) ;
#20897=DIRECTION ( 'NONE',  ( 0.7334850928793760216, 0.6768732144311038201, -0.06198604769976983481 ) ) ;
#20918=ORIENTED_EDGE ( 'NONE', *, *, #10124, .T. ) ;
#20919=DIRECTION ( 'NONE',  ( 0.000000000000000000, 1.000000000000000000, 0.000000000000000000 ) ) ;
#20920=AXIS2_PLACEMENT_3D ( 'NONE', #8425, #4902, #20139 ) ;
#20922=CARTESIAN_POINT ( 'NONE',  ( 59.61686353177688602, 34.52875999999999834, -0.7993558564620834028 ) ) ;
#20930=ORIENTED_EDGE ( 'NONE', *, *, #13217, .T. ) ;
#20932=DIRECTION ( 'NONE',  ( 0.000000000000000000, 1.000000000000000000, 0.000000000000000000 ) ) ;
#20936=ADVANCED_FACE ( 'NONE', ( #3987 ), #7300, .F. ) ;
#20943=DIRECTION ( 'NONE',  ( 0.08420877549337302259, 0.000000000000000000, 0.9964481331860212121 ) ) ;
#20955=AXIS2_PLACEMENT_3D ( 'NONE', #14924, #11688, #8260 ) ;
#20974=ORIENTED_EDGE ( 'NONE', *, *, #18022, .F. ) ;
#20975=LINE ( 'NONE', #8799, #5070 ) ;
#21003=ORIENTED_EDGE ( 'NONE', *, *, #19137, .F. ) ;
#21010=EDGE_CURVE ( 'NONE', #10479, #20861, #16685, .T. ) ;
#21012=DIRECTION ( 'NONE',  ( -0.2672484743474500268, 0.000000000000000000, -0.9636276526537417286 ) ) ;
#21022=DIRECTION ( 'NONE',  ( 0.000000000000000000, 1.000000000000000000, 0.000000000000000000 ) ) ;
#21027=CARTESIAN_POINT ( 'NONE',  ( 9.256853431388732290, 34.52875999999999834, -17.09316853730597074 ) ) ;
#21028=DIRECTION ( 'NONE',  ( 0.000000000000000000, 1.000000000000000000, 0.000000000000000000 ) ) ;
#21030=EDGE_LOOP ( 'NONE', ( #8836, #21780, #6727, #4727 ) ) ;
#21033=ORIENTED_EDGE ( 'NONE', *, *, #8412, .F. ) ;
#21040=CARTESIAN_POINT ( 'NONE',  ( 28.56548256563643662, -3.968114999999999615, -12.12873025803960658 ) ) ;
#21044=VERTEX_POINT ( 'NONE', #18009 ) ;
#21052=DIRECTION ( 'NONE',  ( 0.000000000000000000, 1.000000000000000000, 0.000000000000000000 ) ) ;
#21070=AXIS2_PLACEMENT_3D ( 'NONE', #8538, #16745, #16842 ) ;
#21072=ORIENTED_EDGE ( 'NONE', *, *, #2720, .F. ) ;
#21073=CARTESIAN_POINT ( 'NONE',  ( 12.25799425556778388, 34.52875999999999834, 0.2069032437451798767 ) ) ;
#21078=EDGE_CURVE ( 'NONE', #337, #6373, #5741, .T. ) ;
#21087=VERTEX_POINT ( 'NONE', #9601 ) ;
#21096=CARTESIAN_POINT ( 'NONE',  ( 19.79515554403045741, 34.52875999999999834, -10.69562145279641996 ) ) ;
#21098=DIRECTION ( 'NONE',  ( -0.9173788132826627972, 0.000000000000000000, 0.3980152169705239440 ) ) ;
#21103=EDGE_CURVE ( 'NONE', #10784, #8462, #9615, .T. ) ;
#21104=LINE ( 'NONE', #5955, #16493 ) ;
#21107=VERTEX_POINT ( 'NONE', #4279 ) ;
#21115=DIRECTION ( 'NONE',  ( 0.08420877549337300871, 0.000000000000000000, 0.9964481331860212121 ) ) ;
#21116=CARTESIAN_POINT ( 'NONE',  ( -40.81626320044254896, 38.26001999999999725, 60.06868603633916592 ) ) ;
#21119=DIRECTION ( 'NONE',  ( 0.000000000000000000, 1.000000000000000000, 0.000000000000000000 ) ) ;
#21128=ORIENTED_EDGE ( 'NONE', *, *, #2516, .T. ) ;
#21129=CARTESIAN_POINT ( 'NONE',  ( 55.81697695389291169, -3.968114999999999615, -11.14520323105768362 ) ) ;
#21136=LINE ( 'NONE', #21040, #11628 ) ;
#21160=CARTESIAN_POINT ( 'NONE',  ( 46.03750000000000142, -1.983739999999999393, -10.31874999999999964 ) ) ;
#21170=CARTESIAN_POINT ( 'NONE',  ( 66.79943102505561114, -3.968114999999999615, -12.07331878313145168 ) ) ;
#21171=AXIS2_PLACEMENT_3D ( 'NONE', #20564, #14193, #10956 ) ;
#21182=CARTESIAN_POINT ( 'NONE',  ( 46.03750000000000142, -14.84248999999999974, -10.31874999999999964 ) ) ;
#21187=CARTESIAN_POINT ( 'NONE',  ( 46.03750000000000142, 34.52875999999999834, -10.31874999999999964 ) ) ;
#21194=EDGE_LOOP ( 'NONE', ( #9583, #8628, #1662, #14921 ) ) ;
#21195=VECTOR ( 'NONE', #5244, 1000.000000000000114 ) ;
#21197=EDGE_CURVE ( 'NONE', #21087, #11237, #6793, .T. ) ;
#21200=DIRECTION ( 'NONE',  ( 0.000000000000000000, 1.000000000000000000, 0.000000000000000000 ) ) ;
#21214=CARTESIAN_POINT ( 'NONE',  ( -47.86049599909252805, 41.43438499999999891, -23.29373766372935961 ) ) ;
#21224=VECTOR ( 'NONE', #7582, 1000.000000000000000 ) ;
#21242=CARTESIAN_POINT ( 'NONE',  ( 17.79723720954694954, 34.52875999999999834, -14.07647485258271303 ) ) ;
#21254=VERTEX_POINT ( 'NONE', #12470 ) ;
#21263=LINE ( 'NONE', #19496, #10346 ) ;
#21264=LINE ( 'NONE', #16518, #18174 ) ;
#21269=DIRECTION ( 'NONE',  ( 0.000000000000000000, 1.000000000000000000, 0.000000000000000000 ) ) ;
#21270=DIRECTION ( 'NONE',  ( -0.2672484743474500268, 0.000000000000000000, -0.9636276526537417286 ) ) ;
#21282=CIRCLE ( 'NONE', #11756, 20.83593750000000000 ) ;
#21286=DIRECTION ( 'NONE',  ( -9.174536502825477718E-16, 1.000000000000000000, -1.085629106648973872E-14 ) ) ;
#21307=VERTEX_POINT ( 'NONE', #2592 ) ;
#21309=EDGE_LOOP ( 'NONE', ( #8336, #5822, #10489, #14751 ) ) ;
#21316=ORIENTED_EDGE ( 'NONE', *, *, #18409, .T. ) ;
#21317=CARTESIAN_POINT ( 'NONE',  ( -51.69815163306579819, 38.26001999999999725, -7.436124251198355850 ) ) ;
#21327=AXIS2_PLACEMENT_3D ( 'NONE', #17900, #2748, #9482 ) ;
#21329=ORIENTED_EDGE ( 'NONE', *, *, #11517, .T. ) ;
#21338=DIRECTION ( 'NONE',  ( -0.9636276526537417286, 0.000000000000000000, 0.2672484743474501934 ) ) ;
#21344=CARTESIAN_POINT ( 'NONE',  ( -15.27766260488554195, 34.52875999999999834, -26.04727837583638461 ) ) ;
#21357=VERTEX_POINT ( 'NONE', #12444 ) ;
#21362=ORIENTED_EDGE ( 'NONE', *, *, #16309, .T. ) ;
#21374=ORIENTED_EDGE ( 'NONE', *, *, #8671, .T. ) ;
#21381=DIRECTION ( 'NONE',  ( 0.000000000000000000, 1.000000000000000000, 0.000000000000000000 ) ) ;
#21385=CARTESIAN_POINT ( 'NONE',  ( -28.19602381335591801, 39.45064500000000152, -72.46697370030818774 ) ) ;
#21386=VERTEX_POINT ( 'NONE', #8885 ) ;
#21388=CARTESIAN_POINT ( 'NONE',  ( 36.54633153140315471, -14.84248999999999974, -9.516661413425623550 ) ) ;
#21397=ADVANCED_FACE ( 'NONE', ( #601 ), #14111, .F. ) ;
#21401=FACE_OUTER_BOUND ( 'NONE', #6681, .T. ) ;
#21404=ORIENTED_EDGE ( 'NONE', *, *, #12684, .F. ) ;
#21411=ORIENTED_EDGE ( 'NONE', *, *, #6799, .F. ) ;
#21413=AXIS2_PLACEMENT_3D ( 'NONE', #8102, #19507, #9549 ) ;
#21418=FACE_OUTER_BOUND ( 'NONE', #5119, .T. ) ;
#21424=EDGE_LOOP ( 'NONE', ( #6638, #3159, #8630, #2301, #17450, #4838, #4127, #1633, #1855, #17533, #4297, #16782, #3807, #21743, #16666, #17563, #15918, #919, #16915, #13967, #5155, #14852 ) ) ;
#21430=EDGE_LOOP ( 'NONE', ( #15780, #4086, #6723, #17150, #828 ) ) ;
#21440=CARTESIAN_POINT ( 'NONE',  ( -15.41509608936259035, 37.15413452960619622, -10.31276839742836415 ) ) ;
#21445=EDGE_CURVE ( 'NONE', #6011, #18301, #4688, .T. ) ;
#21478=ORIENTED_EDGE ( 'NONE', *, *, #6927, .F. ) ;
#21481=EDGE_CURVE ( 'NONE', #8950, #21616, #21263, .T. ) ;
#21482=VERTEX_POINT ( 'NONE', #4797 ) ;
#21485=CARTESIAN_POINT ( 'NONE',  ( 44.28293121686854761, -1.983739999999999393, -31.08068102505560759 ) ) ;
#21494=ORIENTED_EDGE ( 'NONE', *, *, #17921, .F. ) ;
#21508=CYLINDRICAL_SURFACE ( 'NONE', #2596, 0.7950200000000000600 ) ;
#21518=VECTOR ( 'NONE', #18061, 1000.000000000000000 ) ;
#21527=LINE ( 'NONE', #13156, #54 ) ;
#21530=DIRECTION ( 'NONE',  ( -0.000000000000000000, -1.000000000000000000, 0.000000000000000000 ) ) ;
#21533=CARTESIAN_POINT ( 'NONE',  ( 28.56548256563643662, 34.52875999999999834, -12.12873025803960658 ) ) ;
#21537=EDGE_CURVE ( 'NONE', #6939, #16850, #21644, .T. ) ;
#21554=DIRECTION ( 'NONE',  ( -9.174536502825477718E-16, 1.000000000000000000, -1.085629106648973872E-14 ) ) ;
#21576=VECTOR ( 'NONE', #3261, 1000.000000000000000 ) ;
#21578=CARTESIAN_POINT ( 'NONE',  ( 30.42699695299585017, 34.52875999999999834, -4.832012189960551041 ) ) ;
#21581=AXIS2_PLACEMENT_3D ( 'NONE', #21129, #5981, #2686 ) ;
#21601=( BOUNDED_CURVE ( )  B_SPLINE_CURVE ( 3, ( #7275, #11107, #17330, #17860 ),
 .UNSPECIFIED., .F., .T. ) 
 B_SPLINE_CURVE_WITH_KNOTS ( ( 4, 4 ),
 ( 1.199226304266461929, 1.570796326795209863 ),
 .UNSPECIFIED. ) 
 CURVE ( )  GEOMETRIC_REPRESENTATION_ITEM ( )  RATIONAL_B_SPLINE_CURVE ( ( 1.000000000000000000, 0.9885276984537190170, 0.9885276984537190170, 1.000000000000000000 ) ) 
 REPRESENTATION_ITEM ( '' )  );
#21611=CARTESIAN_POINT ( 'NONE',  ( 11.82678039945931481, -3.968114999999999615, -12.74436900065013667 ) ) ;
#21612=AXIS2_PLACEMENT_3D ( 'NONE', #9932, #9819, #15051 ) ;
#21613=VERTEX_POINT ( 'NONE', #18587 ) ;
#21616=VERTEX_POINT ( 'NONE', #11635 ) ;
#21627=VERTEX_POINT ( 'NONE', #8211 ) ;
#21630=CARTESIAN_POINT ( 'NONE',  ( 9.828862065001116477, -1.983739999999999393, -16.12522240043857025 ) ) ;
#21637=EDGE_CURVE ( 'NONE', #19617, #1298, #14967, .T. ) ;
#21644=CIRCLE ( 'NONE', #3643, 9.524999999999996803 ) ;
#21649=ORIENTED_EDGE ( 'NONE', *, *, #21637, .T. ) ;
#21650=DIRECTION ( 'NONE',  ( 0.000000000000000000, 1.000000000000000000, 0.000000000000000000 ) ) ;
#21651=DIRECTION ( 'NONE',  ( 0.3447671952293626108, 0.000000000000000000, 0.9386882235831439658 ) ) ;
#21661=ORIENTED_EDGE ( 'NONE', *, *, #13479, .T. ) ;
#21664=AXIS2_PLACEMENT_3D ( 'NONE', #15633, #15846, #14079 ) ;
#21668=CIRCLE ( 'NONE', #15350, 0.3962400000000000366 ) ;
#21673=DIRECTION ( 'NONE',  ( 0.08420877549337300871, 0.000000000000000000, 0.9964481331860212121 ) ) ;
#21684=LINE ( 'NONE', #10070, #3954 ) ;
#21695=CIRCLE ( 'NONE', #14304, 1.191259999999998209 ) ;
#21719=DIRECTION ( 'NONE',  ( 0.08420877549337300871, 0.000000000000000000, 0.9964481331860212121 ) ) ;
#21720=ORIENTED_EDGE ( 'NONE', *, *, #9813, .T. ) ;
#21724=ORIENTED_EDGE ( 'NONE', *, *, #3867, .F. ) ;
#21733=EDGE_CURVE ( 'NONE', #11228, #1298, #14986, .T. ) ;
#21739=VERTEX_POINT ( 'NONE', #3358 ) ;
#21743=ORIENTED_EDGE ( 'NONE', *, *, #14166, .T. ) ;
#21754=EDGE_CURVE ( 'NONE', #21107, #10001, #8917, .T. ) ;
#21763=CARTESIAN_POINT ( 'NONE',  ( 12.38912331111999343, -14.84248999999999974, 5.137219823516766759 ) ) ;
#21772=DIRECTION ( 'NONE',  ( 0.000000000000000000, 1.000000000000000000, 0.000000000000000000 ) ) ;
#21777=CARTESIAN_POINT ( 'NONE',  ( -24.20935654380574320, 41.43438499999999891, -25.29247038871795894 ) ) ;
#21780=ORIENTED_EDGE ( 'NONE', *, *, #4617, .F. ) ;
#21786=EDGE_LOOP ( 'NONE', ( #10905, #2632, #6948, #11138, #2961, #5928 ) ) ;
#21796=EDGE_CURVE ( 'NONE', #6011, #19768, #13529, .T. ) ;
#21798=CARTESIAN_POINT ( 'NONE',  ( -15.40073180542343501, -4.594366328436724878, -10.30507461945350833 ) ) ;
#21809=CARTESIAN_POINT ( 'NONE',  ( 17.22522857595987844, -1.983739999999999393, -15.04442098945225403 ) ) ;
#21825=EDGE_CURVE ( 'NONE', #11084, #11404, #20790, .T. ) ;
#21827=AXIS2_PLACEMENT_3D ( 'NONE', #10462, #18631, #10566 ) ;
#21832=CARTESIAN_POINT ( 'NONE',  ( -21.29909891687151813, 42.13594019876639862, -25.53841317587618320 ) ) ;
#21835=PRODUCT_DEFINITION_CONTEXT ( 'detailed design', #19766, 'design' ) ;
#21841=ORIENTED_EDGE ( 'NONE', *, *, #12438, .F. ) ;
#21847=ORIENTED_EDGE ( 'NONE', *, *, #20309, .T. ) ;
#21858=CARTESIAN_POINT ( 'NONE',  ( -51.02421882195815783, 38.25938500000000175, -23.02637480153789795 ) ) ;
#21867=CARTESIAN_POINT ( 'NONE',  ( -51.69815163306579819, -14.84248999999999974, -7.436124251198355850 ) ) ;
#21882=DIRECTION ( 'NONE',  ( 0.000000000000000000, -1.000000000000000000, 0.000000000000000000 ) ) ;
ENDSEC;
END-ISO-10303-21;
